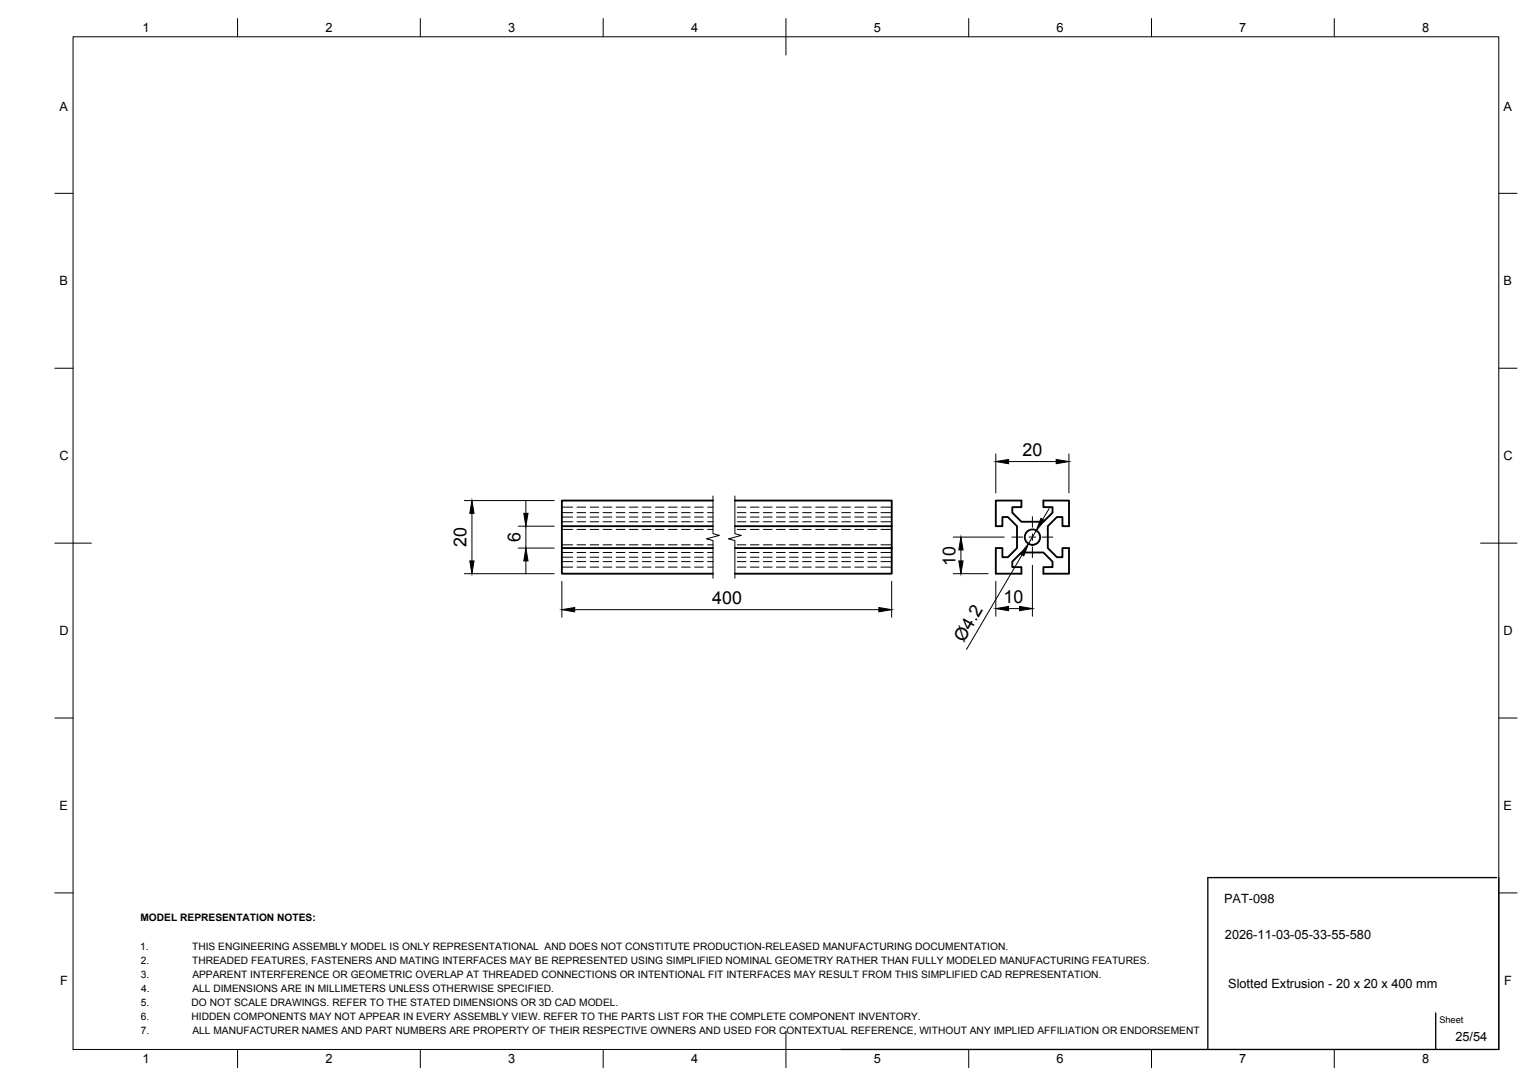
ISO-10303-21;
HEADER;
/* Generated by software containing ST-Developer
 * from STEP Tools, Inc. (www.steptools.com) 
 */

FILE_DESCRIPTION(
/* description */ ('Spring compression tester'),
/* implementation_level */ '2;1');

FILE_NAME(
/* name */ 'Slotted Extrusion - 20 x 20 x 400 mm.step',
/* time_stamp */ '2026-10-28T03:24:11-07:00',
/* author */ (''),
/* organization */ (''),
/* preprocessor_version */ 'ST-DEVELOPER v20.2',
/* originating_system */ 'Autodesk Translation Framework v15.17.0.0',
/* authorisation */ '');

FILE_SCHEMA (('AUTOMOTIVE_DESIGN { 1 0 10303 214 3 1 1 }'));
ENDSEC;

DATA;
#10=MECHANICAL_DESIGN_GEOMETRIC_PRESENTATION_REPRESENTATION('',(#1154),#43521);
#1019=SHAPE_REPRESENTATION_RELATIONSHIP('SRR','None',#43833,#1079);
#1079=ADVANCED_BREP_SHAPE_REPRESENTATION('',(#1226),#43493);
#1154=STYLED_ITEM('',(#44188),#1226);
#1226=MANIFOLD_SOLID_BREP('Body1',#18594);
#1471=FACE_BOUND('',#4046,.T.);
#1472=FACE_BOUND('',#4048,.T.);
#1944=PLANE('',#20307);
#1945=PLANE('',#20308);
#1946=PLANE('',#20309);
#1947=PLANE('',#20310);
#1948=PLANE('',#20311);
#1949=PLANE('',#20312);
#1950=PLANE('',#20313);
#1951=PLANE('',#20314);
#1952=PLANE('',#20315);
#1953=PLANE('',#20316);
#1954=PLANE('',#20317);
#1955=PLANE('',#20318);
#1956=PLANE('',#20319);
#1957=PLANE('',#20320);
#1958=PLANE('',#20321);
#1959=PLANE('',#20322);
#1960=PLANE('',#20323);
#1961=PLANE('',#20324);
#1962=PLANE('',#20325);
#1963=PLANE('',#20326);
#1964=PLANE('',#20327);
#1965=PLANE('',#20328);
#1966=PLANE('',#20329);
#1967=PLANE('',#20330);
#1968=PLANE('',#20331);
#1969=PLANE('',#20332);
#1970=PLANE('',#20333);
#1971=PLANE('',#20334);
#1972=PLANE('',#20335);
#1973=PLANE('',#20336);
#1974=PLANE('',#20337);
#1975=PLANE('',#20338);
#1976=PLANE('',#20339);
#1977=PLANE('',#20340);
#1978=PLANE('',#20341);
#1979=PLANE('',#20342);
#1980=PLANE('',#20346);
#1981=PLANE('',#20347);
#1982=PLANE('',#20348);
#1983=PLANE('',#20349);
#1984=PLANE('',#20350);
#1985=PLANE('',#20351);
#1986=PLANE('',#20352);
#1987=PLANE('',#20353);
#1988=PLANE('',#20354);
#1989=PLANE('',#20355);
#2729=FACE_OUTER_BOUND('',#4000,.T.);
#2730=FACE_OUTER_BOUND('',#4001,.T.);
#2731=FACE_OUTER_BOUND('',#4002,.T.);
#2732=FACE_OUTER_BOUND('',#4003,.T.);
#2733=FACE_OUTER_BOUND('',#4004,.T.);
#2734=FACE_OUTER_BOUND('',#4005,.T.);
#2735=FACE_OUTER_BOUND('',#4006,.T.);
#2736=FACE_OUTER_BOUND('',#4007,.T.);
#2737=FACE_OUTER_BOUND('',#4008,.T.);
#2738=FACE_OUTER_BOUND('',#4009,.T.);
#2739=FACE_OUTER_BOUND('',#4010,.T.);
#2740=FACE_OUTER_BOUND('',#4011,.T.);
#2741=FACE_OUTER_BOUND('',#4012,.T.);
#2742=FACE_OUTER_BOUND('',#4013,.T.);
#2743=FACE_OUTER_BOUND('',#4014,.T.);
#2744=FACE_OUTER_BOUND('',#4015,.T.);
#2745=FACE_OUTER_BOUND('',#4016,.T.);
#2746=FACE_OUTER_BOUND('',#4017,.T.);
#2747=FACE_OUTER_BOUND('',#4018,.T.);
#2748=FACE_OUTER_BOUND('',#4019,.T.);
#2749=FACE_OUTER_BOUND('',#4020,.T.);
#2750=FACE_OUTER_BOUND('',#4021,.T.);
#2751=FACE_OUTER_BOUND('',#4022,.T.);
#2752=FACE_OUTER_BOUND('',#4023,.T.);
#2753=FACE_OUTER_BOUND('',#4024,.T.);
#2754=FACE_OUTER_BOUND('',#4025,.T.);
#2755=FACE_OUTER_BOUND('',#4026,.T.);
#2756=FACE_OUTER_BOUND('',#4027,.T.);
#2757=FACE_OUTER_BOUND('',#4028,.T.);
#2758=FACE_OUTER_BOUND('',#4029,.T.);
#2759=FACE_OUTER_BOUND('',#4030,.T.);
#2760=FACE_OUTER_BOUND('',#4031,.T.);
#2761=FACE_OUTER_BOUND('',#4032,.T.);
#2762=FACE_OUTER_BOUND('',#4033,.T.);
#2763=FACE_OUTER_BOUND('',#4034,.T.);
#2764=FACE_OUTER_BOUND('',#4035,.T.);
#2765=FACE_OUTER_BOUND('',#4036,.T.);
#2766=FACE_OUTER_BOUND('',#4037,.T.);
#2767=FACE_OUTER_BOUND('',#4038,.T.);
#2768=FACE_OUTER_BOUND('',#4039,.T.);
#2769=FACE_OUTER_BOUND('',#4040,.T.);
#2770=FACE_OUTER_BOUND('',#4041,.T.);
#2771=FACE_OUTER_BOUND('',#4042,.T.);
#2772=FACE_OUTER_BOUND('',#4043,.T.);
#2773=FACE_OUTER_BOUND('',#4044,.T.);
#2774=FACE_OUTER_BOUND('',#4045,.T.);
#2775=FACE_OUTER_BOUND('',#4047,.T.);
#4000=EDGE_LOOP('',(#14657,#14658,#14659,#14660));
#4001=EDGE_LOOP('',(#14661,#14662,#14663,#14664));
#4002=EDGE_LOOP('',(#14665,#14666,#14667,#14668));
#4003=EDGE_LOOP('',(#14669,#14670,#14671,#14672));
#4004=EDGE_LOOP('',(#14673,#14674,#14675,#14676));
#4005=EDGE_LOOP('',(#14677,#14678,#14679,#14680));
#4006=EDGE_LOOP('',(#14681,#14682,#14683,#14684));
#4007=EDGE_LOOP('',(#14685,#14686,#14687,#14688));
#4008=EDGE_LOOP('',(#14689,#14690,#14691,#14692));
#4009=EDGE_LOOP('',(#14693,#14694,#14695,#14696));
#4010=EDGE_LOOP('',(#14697,#14698,#14699,#14700));
#4011=EDGE_LOOP('',(#14701,#14702,#14703,#14704));
#4012=EDGE_LOOP('',(#14705,#14706,#14707,#14708));
#4013=EDGE_LOOP('',(#14709,#14710,#14711,#14712));
#4014=EDGE_LOOP('',(#14713,#14714,#14715,#14716));
#4015=EDGE_LOOP('',(#14717,#14718,#14719,#14720));
#4016=EDGE_LOOP('',(#14721,#14722,#14723,#14724));
#4017=EDGE_LOOP('',(#14725,#14726,#14727,#14728));
#4018=EDGE_LOOP('',(#14729,#14730,#14731,#14732));
#4019=EDGE_LOOP('',(#14733,#14734,#14735,#14736));
#4020=EDGE_LOOP('',(#14737,#14738,#14739,#14740));
#4021=EDGE_LOOP('',(#14741,#14742,#14743,#14744));
#4022=EDGE_LOOP('',(#14745,#14746,#14747,#14748));
#4023=EDGE_LOOP('',(#14749,#14750,#14751,#14752));
#4024=EDGE_LOOP('',(#14753,#14754,#14755,#14756));
#4025=EDGE_LOOP('',(#14757,#14758,#14759,#14760));
#4026=EDGE_LOOP('',(#14761,#14762,#14763,#14764));
#4027=EDGE_LOOP('',(#14765,#14766,#14767,#14768));
#4028=EDGE_LOOP('',(#14769,#14770,#14771,#14772));
#4029=EDGE_LOOP('',(#14773,#14774,#14775,#14776));
#4030=EDGE_LOOP('',(#14777,#14778,#14779,#14780));
#4031=EDGE_LOOP('',(#14781,#14782,#14783,#14784));
#4032=EDGE_LOOP('',(#14785,#14786,#14787,#14788));
#4033=EDGE_LOOP('',(#14789,#14790,#14791,#14792));
#4034=EDGE_LOOP('',(#14793,#14794,#14795,#14796));
#4035=EDGE_LOOP('',(#14797,#14798,#14799,#14800));
#4036=EDGE_LOOP('',(#14801,#14802,#14803,#14804));
#4037=EDGE_LOOP('',(#14805,#14806,#14807,#14808));
#4038=EDGE_LOOP('',(#14809,#14810,#14811,#14812));
#4039=EDGE_LOOP('',(#14813,#14814,#14815,#14816));
#4040=EDGE_LOOP('',(#14817,#14818,#14819,#14820));
#4041=EDGE_LOOP('',(#14821,#14822,#14823,#14824));
#4042=EDGE_LOOP('',(#14825,#14826,#14827,#14828));
#4043=EDGE_LOOP('',(#14829,#14830,#14831,#14832));
#4044=EDGE_LOOP('',(#14833,#14834,#14835,#14836));
#4045=EDGE_LOOP('',(#14837,#14838,#14839,#14840,#14841,#14842,#14843,#14844,
#14845,#14846,#14847,#14848,#14849,#14850,#14851,#14852,#14853,#14854,#14855,
#14856,#14857,#14858,#14859,#14860,#14861,#14862,#14863,#14864,#14865,#14866,
#14867,#14868,#14869,#14870,#14871,#14872,#14873,#14874,#14875,#14876,#14877,
#14878,#14879,#14880));
#4046=EDGE_LOOP('',(#14881));
#4047=EDGE_LOOP('',(#14882,#14883,#14884,#14885,#14886,#14887,#14888,#14889,
#14890,#14891,#14892,#14893,#14894,#14895,#14896,#14897,#14898,#14899,#14900,
#14901,#14902,#14903,#14904,#14905,#14906,#14907,#14908,#14909,#14910,#14911,
#14912,#14913,#14914,#14915,#14916,#14917,#14918,#14919,#14920,#14921,#14922,
#14923,#14924,#14925));
#4048=EDGE_LOOP('',(#14926));
#5380=LINE('',#29743,#6812);
#5381=LINE('',#29745,#6813);
#5382=LINE('',#29747,#6814);
#5383=LINE('',#29748,#6815);
#5384=LINE('',#29751,#6816);
#5385=LINE('',#29753,#6817);
#5386=LINE('',#29754,#6818);
#5387=LINE('',#29757,#6819);
#5388=LINE('',#29759,#6820);
#5389=LINE('',#29760,#6821);
#5390=LINE('',#29763,#6822);
#5391=LINE('',#29765,#6823);
#5392=LINE('',#29766,#6824);
#5393=LINE('',#29769,#6825);
#5394=LINE('',#29771,#6826);
#5395=LINE('',#29772,#6827);
#5396=LINE('',#29775,#6828);
#5397=LINE('',#29777,#6829);
#5398=LINE('',#29778,#6830);
#5399=LINE('',#29781,#6831);
#5400=LINE('',#29783,#6832);
#5401=LINE('',#29784,#6833);
#5402=LINE('',#29787,#6834);
#5403=LINE('',#29789,#6835);
#5404=LINE('',#29790,#6836);
#5405=LINE('',#29793,#6837);
#5406=LINE('',#29795,#6838);
#5407=LINE('',#29796,#6839);
#5408=LINE('',#29800,#6840);
#5409=LINE('',#29802,#6841);
#5410=LINE('',#29804,#6842);
#5411=LINE('',#29805,#6843);
#5412=LINE('',#29808,#6844);
#5413=LINE('',#29810,#6845);
#5414=LINE('',#29811,#6846);
#5415=LINE('',#29814,#6847);
#5416=LINE('',#29816,#6848);
#5417=LINE('',#29817,#6849);
#5418=LINE('',#29820,#6850);
#5419=LINE('',#29822,#6851);
#5420=LINE('',#29823,#6852);
#5421=LINE('',#29826,#6853);
#5422=LINE('',#29828,#6854);
#5423=LINE('',#29829,#6855);
#5424=LINE('',#29832,#6856);
#5425=LINE('',#29834,#6857);
#5426=LINE('',#29835,#6858);
#5427=LINE('',#29838,#6859);
#5428=LINE('',#29840,#6860);
#5429=LINE('',#29841,#6861);
#5430=LINE('',#29844,#6862);
#5431=LINE('',#29846,#6863);
#5432=LINE('',#29847,#6864);
#5433=LINE('',#29850,#6865);
#5434=LINE('',#29852,#6866);
#5435=LINE('',#29853,#6867);
#5436=LINE('',#29857,#6868);
#5437=LINE('',#29859,#6869);
#5438=LINE('',#29861,#6870);
#5439=LINE('',#29862,#6871);
#5440=LINE('',#29865,#6872);
#5441=LINE('',#29867,#6873);
#5442=LINE('',#29868,#6874);
#5443=LINE('',#29871,#6875);
#5444=LINE('',#29873,#6876);
#5445=LINE('',#29874,#6877);
#5446=LINE('',#29877,#6878);
#5447=LINE('',#29879,#6879);
#5448=LINE('',#29880,#6880);
#5449=LINE('',#29883,#6881);
#5450=LINE('',#29885,#6882);
#5451=LINE('',#29886,#6883);
#5452=LINE('',#29889,#6884);
#5453=LINE('',#29891,#6885);
#5454=LINE('',#29892,#6886);
#5455=LINE('',#29895,#6887);
#5456=LINE('',#29897,#6888);
#5457=LINE('',#29898,#6889);
#5458=LINE('',#29901,#6890);
#5459=LINE('',#29903,#6891);
#5460=LINE('',#29904,#6892);
#5461=LINE('',#29907,#6893);
#5462=LINE('',#29909,#6894);
#5463=LINE('',#29910,#6895);
#5464=LINE('',#29914,#6896);
#5465=LINE('',#29916,#6897);
#5466=LINE('',#29918,#6898);
#5467=LINE('',#29919,#6899);
#5468=LINE('',#29922,#6900);
#5469=LINE('',#29924,#6901);
#5470=LINE('',#29925,#6902);
#5471=LINE('',#29928,#6903);
#5472=LINE('',#29930,#6904);
#5473=LINE('',#29931,#6905);
#5474=LINE('',#29934,#6906);
#5475=LINE('',#29936,#6907);
#5476=LINE('',#29937,#6908);
#5477=LINE('',#29940,#6909);
#5478=LINE('',#29942,#6910);
#5479=LINE('',#29943,#6911);
#5480=LINE('',#29946,#6912);
#5481=LINE('',#29948,#6913);
#5482=LINE('',#29949,#6914);
#5483=LINE('',#29952,#6915);
#5484=LINE('',#29954,#6916);
#5485=LINE('',#29955,#6917);
#5486=LINE('',#29958,#6918);
#5487=LINE('',#29960,#6919);
#5488=LINE('',#29961,#6920);
#5489=LINE('',#29964,#6921);
#5490=LINE('',#29966,#6922);
#5491=LINE('',#29967,#6923);
#5492=LINE('',#29972,#6924);
#5493=LINE('',#29976,#6925);
#5494=LINE('',#29978,#6926);
#5495=LINE('',#29979,#6927);
#5496=LINE('',#29982,#6928);
#5497=LINE('',#29984,#6929);
#5498=LINE('',#29985,#6930);
#5499=LINE('',#29987,#6931);
#5500=LINE('',#29988,#6932);
#5501=LINE('',#29991,#6933);
#5502=LINE('',#29993,#6934);
#5503=LINE('',#29994,#6935);
#5504=LINE('',#29996,#6936);
#5505=LINE('',#29997,#6937);
#5506=LINE('',#30000,#6938);
#5507=LINE('',#30002,#6939);
#5508=LINE('',#30003,#6940);
#5509=LINE('',#30005,#6941);
#5510=LINE('',#30006,#6942);
#5511=LINE('',#30008,#6943);
#5512=LINE('',#30009,#6944);
#6812=VECTOR('',#24018,1.);
#6813=VECTOR('',#24019,1.);
#6814=VECTOR('',#24020,1.);
#6815=VECTOR('',#24021,1.);
#6816=VECTOR('',#24024,1.);
#6817=VECTOR('',#24025,1.);
#6818=VECTOR('',#24026,1.);
#6819=VECTOR('',#24029,1.);
#6820=VECTOR('',#24030,1.);
#6821=VECTOR('',#24031,1.);
#6822=VECTOR('',#24034,1.);
#6823=VECTOR('',#24035,1.);
#6824=VECTOR('',#24036,1.);
#6825=VECTOR('',#24039,1.);
#6826=VECTOR('',#24040,1.);
#6827=VECTOR('',#24041,1.);
#6828=VECTOR('',#24044,1.);
#6829=VECTOR('',#24045,1.);
#6830=VECTOR('',#24046,1.);
#6831=VECTOR('',#24049,1.);
#6832=VECTOR('',#24050,1.);
#6833=VECTOR('',#24051,1.);
#6834=VECTOR('',#24054,1.);
#6835=VECTOR('',#24055,1.);
#6836=VECTOR('',#24056,1.);
#6837=VECTOR('',#24059,1.);
#6838=VECTOR('',#24060,1.);
#6839=VECTOR('',#24061,1.);
#6840=VECTOR('',#24064,1.);
#6841=VECTOR('',#24065,1.);
#6842=VECTOR('',#24066,1.);
#6843=VECTOR('',#24067,1.);
#6844=VECTOR('',#24070,1.);
#6845=VECTOR('',#24071,1.);
#6846=VECTOR('',#24072,1.);
#6847=VECTOR('',#24075,1.);
#6848=VECTOR('',#24076,1.);
#6849=VECTOR('',#24077,1.);
#6850=VECTOR('',#24080,1.);
#6851=VECTOR('',#24081,1.);
#6852=VECTOR('',#24082,1.);
#6853=VECTOR('',#24085,1.);
#6854=VECTOR('',#24086,1.);
#6855=VECTOR('',#24087,1.);
#6856=VECTOR('',#24090,1.);
#6857=VECTOR('',#24091,1.);
#6858=VECTOR('',#24092,1.);
#6859=VECTOR('',#24095,1.);
#6860=VECTOR('',#24096,1.);
#6861=VECTOR('',#24097,1.);
#6862=VECTOR('',#24100,1.);
#6863=VECTOR('',#24101,1.);
#6864=VECTOR('',#24102,1.);
#6865=VECTOR('',#24105,1.);
#6866=VECTOR('',#24106,1.);
#6867=VECTOR('',#24107,1.);
#6868=VECTOR('',#24110,1.);
#6869=VECTOR('',#24111,1.);
#6870=VECTOR('',#24112,1.);
#6871=VECTOR('',#24113,1.);
#6872=VECTOR('',#24116,1.);
#6873=VECTOR('',#24117,1.);
#6874=VECTOR('',#24118,1.);
#6875=VECTOR('',#24121,1.);
#6876=VECTOR('',#24122,1.);
#6877=VECTOR('',#24123,1.);
#6878=VECTOR('',#24126,1.);
#6879=VECTOR('',#24127,1.);
#6880=VECTOR('',#24128,1.);
#6881=VECTOR('',#24131,1.);
#6882=VECTOR('',#24132,1.);
#6883=VECTOR('',#24133,1.);
#6884=VECTOR('',#24136,1.);
#6885=VECTOR('',#24137,1.);
#6886=VECTOR('',#24138,1.);
#6887=VECTOR('',#24141,1.);
#6888=VECTOR('',#24142,1.);
#6889=VECTOR('',#24143,1.);
#6890=VECTOR('',#24146,1.);
#6891=VECTOR('',#24147,1.);
#6892=VECTOR('',#24148,1.);
#6893=VECTOR('',#24151,1.);
#6894=VECTOR('',#24152,1.);
#6895=VECTOR('',#24153,1.);
#6896=VECTOR('',#24156,1.);
#6897=VECTOR('',#24157,1.);
#6898=VECTOR('',#24158,1.);
#6899=VECTOR('',#24159,1.);
#6900=VECTOR('',#24162,1.);
#6901=VECTOR('',#24163,1.);
#6902=VECTOR('',#24164,1.);
#6903=VECTOR('',#24167,1.);
#6904=VECTOR('',#24168,1.);
#6905=VECTOR('',#24169,1.);
#6906=VECTOR('',#24172,1.);
#6907=VECTOR('',#24173,1.);
#6908=VECTOR('',#24174,1.);
#6909=VECTOR('',#24177,1.);
#6910=VECTOR('',#24178,1.);
#6911=VECTOR('',#24179,1.);
#6912=VECTOR('',#24182,1.);
#6913=VECTOR('',#24183,1.);
#6914=VECTOR('',#24184,1.);
#6915=VECTOR('',#24187,1.);
#6916=VECTOR('',#24188,1.);
#6917=VECTOR('',#24189,1.);
#6918=VECTOR('',#24192,1.);
#6919=VECTOR('',#24193,1.);
#6920=VECTOR('',#24194,1.);
#6921=VECTOR('',#24197,1.);
#6922=VECTOR('',#24198,1.);
#6923=VECTOR('',#24199,1.);
#6924=VECTOR('',#24204,0.21);
#6925=VECTOR('',#24209,1.);
#6926=VECTOR('',#24210,1.);
#6927=VECTOR('',#24211,1.);
#6928=VECTOR('',#24214,1.);
#6929=VECTOR('',#24215,1.);
#6930=VECTOR('',#24216,1.);
#6931=VECTOR('',#24219,1.);
#6932=VECTOR('',#24220,1.);
#6933=VECTOR('',#24223,1.);
#6934=VECTOR('',#24224,1.);
#6935=VECTOR('',#24225,1.);
#6936=VECTOR('',#24228,1.);
#6937=VECTOR('',#24229,1.);
#6938=VECTOR('',#24232,1.);
#6939=VECTOR('',#24233,1.);
#6940=VECTOR('',#24234,1.);
#6941=VECTOR('',#24237,1.);
#6942=VECTOR('',#24238,1.);
#6943=VECTOR('',#24241,1.);
#6944=VECTOR('',#24242,1.);
#7884=CIRCLE('',#20344,0.21);
#7885=CIRCLE('',#20345,0.21);
#8963=VERTEX_POINT('',#29741);
#8964=VERTEX_POINT('',#29742);
#8965=VERTEX_POINT('',#29744);
#8966=VERTEX_POINT('',#29746);
#8967=VERTEX_POINT('',#29750);
#8968=VERTEX_POINT('',#29752);
#8969=VERTEX_POINT('',#29756);
#8970=VERTEX_POINT('',#29758);
#8971=VERTEX_POINT('',#29762);
#8972=VERTEX_POINT('',#29764);
#8973=VERTEX_POINT('',#29768);
#8974=VERTEX_POINT('',#29770);
#8975=VERTEX_POINT('',#29774);
#8976=VERTEX_POINT('',#29776);
#8977=VERTEX_POINT('',#29780);
#8978=VERTEX_POINT('',#29782);
#8979=VERTEX_POINT('',#29786);
#8980=VERTEX_POINT('',#29788);
#8981=VERTEX_POINT('',#29792);
#8982=VERTEX_POINT('',#29794);
#8983=VERTEX_POINT('',#29798);
#8984=VERTEX_POINT('',#29799);
#8985=VERTEX_POINT('',#29801);
#8986=VERTEX_POINT('',#29803);
#8987=VERTEX_POINT('',#29807);
#8988=VERTEX_POINT('',#29809);
#8989=VERTEX_POINT('',#29813);
#8990=VERTEX_POINT('',#29815);
#8991=VERTEX_POINT('',#29819);
#8992=VERTEX_POINT('',#29821);
#8993=VERTEX_POINT('',#29825);
#8994=VERTEX_POINT('',#29827);
#8995=VERTEX_POINT('',#29831);
#8996=VERTEX_POINT('',#29833);
#8997=VERTEX_POINT('',#29837);
#8998=VERTEX_POINT('',#29839);
#8999=VERTEX_POINT('',#29843);
#9000=VERTEX_POINT('',#29845);
#9001=VERTEX_POINT('',#29849);
#9002=VERTEX_POINT('',#29851);
#9003=VERTEX_POINT('',#29855);
#9004=VERTEX_POINT('',#29856);
#9005=VERTEX_POINT('',#29858);
#9006=VERTEX_POINT('',#29860);
#9007=VERTEX_POINT('',#29864);
#9008=VERTEX_POINT('',#29866);
#9009=VERTEX_POINT('',#29870);
#9010=VERTEX_POINT('',#29872);
#9011=VERTEX_POINT('',#29876);
#9012=VERTEX_POINT('',#29878);
#9013=VERTEX_POINT('',#29882);
#9014=VERTEX_POINT('',#29884);
#9015=VERTEX_POINT('',#29888);
#9016=VERTEX_POINT('',#29890);
#9017=VERTEX_POINT('',#29894);
#9018=VERTEX_POINT('',#29896);
#9019=VERTEX_POINT('',#29900);
#9020=VERTEX_POINT('',#29902);
#9021=VERTEX_POINT('',#29906);
#9022=VERTEX_POINT('',#29908);
#9023=VERTEX_POINT('',#29912);
#9024=VERTEX_POINT('',#29913);
#9025=VERTEX_POINT('',#29915);
#9026=VERTEX_POINT('',#29917);
#9027=VERTEX_POINT('',#29921);
#9028=VERTEX_POINT('',#29923);
#9029=VERTEX_POINT('',#29927);
#9030=VERTEX_POINT('',#29929);
#9031=VERTEX_POINT('',#29933);
#9032=VERTEX_POINT('',#29935);
#9033=VERTEX_POINT('',#29939);
#9034=VERTEX_POINT('',#29941);
#9035=VERTEX_POINT('',#29945);
#9036=VERTEX_POINT('',#29947);
#9037=VERTEX_POINT('',#29951);
#9038=VERTEX_POINT('',#29953);
#9039=VERTEX_POINT('',#29957);
#9040=VERTEX_POINT('',#29959);
#9041=VERTEX_POINT('',#29963);
#9042=VERTEX_POINT('',#29965);
#9043=VERTEX_POINT('',#29969);
#9044=VERTEX_POINT('',#29971);
#9045=VERTEX_POINT('',#29975);
#9046=VERTEX_POINT('',#29977);
#9047=VERTEX_POINT('',#29981);
#9048=VERTEX_POINT('',#29983);
#9049=VERTEX_POINT('',#29990);
#9050=VERTEX_POINT('',#29992);
#9051=VERTEX_POINT('',#29999);
#9052=VERTEX_POINT('',#30001);
#10993=EDGE_CURVE('',#8963,#8964,#5380,.T.);
#10994=EDGE_CURVE('',#8963,#8965,#5381,.T.);
#10995=EDGE_CURVE('',#8966,#8965,#5382,.T.);
#10996=EDGE_CURVE('',#8964,#8966,#5383,.T.);
#10997=EDGE_CURVE('',#8967,#8963,#5384,.T.);
#10998=EDGE_CURVE('',#8967,#8968,#5385,.T.);
#10999=EDGE_CURVE('',#8965,#8968,#5386,.T.);
#11000=EDGE_CURVE('',#8969,#8967,#5387,.T.);
#11001=EDGE_CURVE('',#8969,#8970,#5388,.T.);
#11002=EDGE_CURVE('',#8968,#8970,#5389,.T.);
#11003=EDGE_CURVE('',#8971,#8969,#5390,.T.);
#11004=EDGE_CURVE('',#8971,#8972,#5391,.T.);
#11005=EDGE_CURVE('',#8970,#8972,#5392,.T.);
#11006=EDGE_CURVE('',#8973,#8971,#5393,.T.);
#11007=EDGE_CURVE('',#8973,#8974,#5394,.T.);
#11008=EDGE_CURVE('',#8972,#8974,#5395,.T.);
#11009=EDGE_CURVE('',#8975,#8973,#5396,.T.);
#11010=EDGE_CURVE('',#8975,#8976,#5397,.T.);
#11011=EDGE_CURVE('',#8974,#8976,#5398,.T.);
#11012=EDGE_CURVE('',#8977,#8975,#5399,.T.);
#11013=EDGE_CURVE('',#8977,#8978,#5400,.T.);
#11014=EDGE_CURVE('',#8976,#8978,#5401,.T.);
#11015=EDGE_CURVE('',#8979,#8977,#5402,.T.);
#11016=EDGE_CURVE('',#8979,#8980,#5403,.T.);
#11017=EDGE_CURVE('',#8978,#8980,#5404,.T.);
#11018=EDGE_CURVE('',#8981,#8979,#5405,.T.);
#11019=EDGE_CURVE('',#8982,#8981,#5406,.T.);
#11020=EDGE_CURVE('',#8980,#8982,#5407,.T.);
#11021=EDGE_CURVE('',#8983,#8984,#5408,.T.);
#11022=EDGE_CURVE('',#8983,#8985,#5409,.T.);
#11023=EDGE_CURVE('',#8986,#8985,#5410,.T.);
#11024=EDGE_CURVE('',#8984,#8986,#5411,.T.);
#11025=EDGE_CURVE('',#8987,#8983,#5412,.T.);
#11026=EDGE_CURVE('',#8987,#8988,#5413,.T.);
#11027=EDGE_CURVE('',#8985,#8988,#5414,.T.);
#11028=EDGE_CURVE('',#8989,#8987,#5415,.T.);
#11029=EDGE_CURVE('',#8989,#8990,#5416,.T.);
#11030=EDGE_CURVE('',#8988,#8990,#5417,.T.);
#11031=EDGE_CURVE('',#8991,#8989,#5418,.T.);
#11032=EDGE_CURVE('',#8991,#8992,#5419,.T.);
#11033=EDGE_CURVE('',#8990,#8992,#5420,.T.);
#11034=EDGE_CURVE('',#8993,#8991,#5421,.T.);
#11035=EDGE_CURVE('',#8993,#8994,#5422,.T.);
#11036=EDGE_CURVE('',#8992,#8994,#5423,.T.);
#11037=EDGE_CURVE('',#8995,#8993,#5424,.T.);
#11038=EDGE_CURVE('',#8995,#8996,#5425,.T.);
#11039=EDGE_CURVE('',#8994,#8996,#5426,.T.);
#11040=EDGE_CURVE('',#8997,#8995,#5427,.T.);
#11041=EDGE_CURVE('',#8997,#8998,#5428,.T.);
#11042=EDGE_CURVE('',#8996,#8998,#5429,.T.);
#11043=EDGE_CURVE('',#8999,#8997,#5430,.T.);
#11044=EDGE_CURVE('',#8999,#9000,#5431,.T.);
#11045=EDGE_CURVE('',#8998,#9000,#5432,.T.);
#11046=EDGE_CURVE('',#9001,#8999,#5433,.T.);
#11047=EDGE_CURVE('',#9002,#9001,#5434,.T.);
#11048=EDGE_CURVE('',#9000,#9002,#5435,.T.);
#11049=EDGE_CURVE('',#9003,#9004,#5436,.T.);
#11050=EDGE_CURVE('',#9003,#9005,#5437,.T.);
#11051=EDGE_CURVE('',#9006,#9005,#5438,.T.);
#11052=EDGE_CURVE('',#9004,#9006,#5439,.T.);
#11053=EDGE_CURVE('',#9007,#9003,#5440,.T.);
#11054=EDGE_CURVE('',#9007,#9008,#5441,.T.);
#11055=EDGE_CURVE('',#9005,#9008,#5442,.T.);
#11056=EDGE_CURVE('',#9009,#9007,#5443,.T.);
#11057=EDGE_CURVE('',#9009,#9010,#5444,.T.);
#11058=EDGE_CURVE('',#9008,#9010,#5445,.T.);
#11059=EDGE_CURVE('',#9011,#9009,#5446,.T.);
#11060=EDGE_CURVE('',#9011,#9012,#5447,.T.);
#11061=EDGE_CURVE('',#9010,#9012,#5448,.T.);
#11062=EDGE_CURVE('',#9013,#9011,#5449,.T.);
#11063=EDGE_CURVE('',#9013,#9014,#5450,.T.);
#11064=EDGE_CURVE('',#9012,#9014,#5451,.T.);
#11065=EDGE_CURVE('',#9015,#9013,#5452,.T.);
#11066=EDGE_CURVE('',#9015,#9016,#5453,.T.);
#11067=EDGE_CURVE('',#9014,#9016,#5454,.T.);
#11068=EDGE_CURVE('',#9017,#9015,#5455,.T.);
#11069=EDGE_CURVE('',#9017,#9018,#5456,.T.);
#11070=EDGE_CURVE('',#9016,#9018,#5457,.T.);
#11071=EDGE_CURVE('',#9019,#9017,#5458,.T.);
#11072=EDGE_CURVE('',#9019,#9020,#5459,.T.);
#11073=EDGE_CURVE('',#9018,#9020,#5460,.T.);
#11074=EDGE_CURVE('',#9021,#9019,#5461,.T.);
#11075=EDGE_CURVE('',#9022,#9021,#5462,.T.);
#11076=EDGE_CURVE('',#9020,#9022,#5463,.T.);
#11077=EDGE_CURVE('',#9023,#9024,#5464,.T.);
#11078=EDGE_CURVE('',#9023,#9025,#5465,.T.);
#11079=EDGE_CURVE('',#9026,#9025,#5466,.T.);
#11080=EDGE_CURVE('',#9024,#9026,#5467,.T.);
#11081=EDGE_CURVE('',#9027,#9023,#5468,.T.);
#11082=EDGE_CURVE('',#9027,#9028,#5469,.T.);
#11083=EDGE_CURVE('',#9025,#9028,#5470,.T.);
#11084=EDGE_CURVE('',#9029,#9027,#5471,.T.);
#11085=EDGE_CURVE('',#9029,#9030,#5472,.T.);
#11086=EDGE_CURVE('',#9028,#9030,#5473,.T.);
#11087=EDGE_CURVE('',#9031,#9029,#5474,.T.);
#11088=EDGE_CURVE('',#9031,#9032,#5475,.T.);
#11089=EDGE_CURVE('',#9030,#9032,#5476,.T.);
#11090=EDGE_CURVE('',#9033,#9031,#5477,.T.);
#11091=EDGE_CURVE('',#9033,#9034,#5478,.T.);
#11092=EDGE_CURVE('',#9032,#9034,#5479,.T.);
#11093=EDGE_CURVE('',#9035,#9033,#5480,.T.);
#11094=EDGE_CURVE('',#9035,#9036,#5481,.T.);
#11095=EDGE_CURVE('',#9034,#9036,#5482,.T.);
#11096=EDGE_CURVE('',#9037,#9035,#5483,.T.);
#11097=EDGE_CURVE('',#9037,#9038,#5484,.T.);
#11098=EDGE_CURVE('',#9036,#9038,#5485,.T.);
#11099=EDGE_CURVE('',#9039,#9037,#5486,.T.);
#11100=EDGE_CURVE('',#9039,#9040,#5487,.T.);
#11101=EDGE_CURVE('',#9038,#9040,#5488,.T.);
#11102=EDGE_CURVE('',#9041,#9039,#5489,.T.);
#11103=EDGE_CURVE('',#9042,#9041,#5490,.T.);
#11104=EDGE_CURVE('',#9040,#9042,#5491,.T.);
#11105=EDGE_CURVE('',#9043,#9043,#7884,.T.);
#11106=EDGE_CURVE('',#9043,#9044,#5492,.T.);
#11107=EDGE_CURVE('',#9044,#9044,#7885,.T.);
#11108=EDGE_CURVE('',#8981,#9045,#5493,.T.);
#11109=EDGE_CURVE('',#9045,#9046,#5494,.T.);
#11110=EDGE_CURVE('',#8982,#9046,#5495,.T.);
#11111=EDGE_CURVE('',#9047,#8966,#5496,.T.);
#11112=EDGE_CURVE('',#9048,#9047,#5497,.T.);
#11113=EDGE_CURVE('',#9048,#8964,#5498,.T.);
#11114=EDGE_CURVE('',#9001,#9048,#5499,.T.);
#11115=EDGE_CURVE('',#9002,#9047,#5500,.T.);
#11116=EDGE_CURVE('',#9049,#8986,#5501,.T.);
#11117=EDGE_CURVE('',#9050,#9049,#5502,.T.);
#11118=EDGE_CURVE('',#9050,#8984,#5503,.T.);
#11119=EDGE_CURVE('',#9021,#9050,#5504,.T.);
#11120=EDGE_CURVE('',#9022,#9049,#5505,.T.);
#11121=EDGE_CURVE('',#9051,#9006,#5506,.T.);
#11122=EDGE_CURVE('',#9052,#9051,#5507,.T.);
#11123=EDGE_CURVE('',#9052,#9004,#5508,.T.);
#11124=EDGE_CURVE('',#9041,#9052,#5509,.T.);
#11125=EDGE_CURVE('',#9042,#9051,#5510,.T.);
#11126=EDGE_CURVE('',#9046,#9026,#5511,.T.);
#11127=EDGE_CURVE('',#9045,#9024,#5512,.T.);
#14657=ORIENTED_EDGE('',*,*,#10993,.F.);
#14658=ORIENTED_EDGE('',*,*,#10994,.T.);
#14659=ORIENTED_EDGE('',*,*,#10995,.F.);
#14660=ORIENTED_EDGE('',*,*,#10996,.F.);
#14661=ORIENTED_EDGE('',*,*,#10997,.F.);
#14662=ORIENTED_EDGE('',*,*,#10998,.T.);
#14663=ORIENTED_EDGE('',*,*,#10999,.F.);
#14664=ORIENTED_EDGE('',*,*,#10994,.F.);
#14665=ORIENTED_EDGE('',*,*,#11000,.F.);
#14666=ORIENTED_EDGE('',*,*,#11001,.T.);
#14667=ORIENTED_EDGE('',*,*,#11002,.F.);
#14668=ORIENTED_EDGE('',*,*,#10998,.F.);
#14669=ORIENTED_EDGE('',*,*,#11003,.F.);
#14670=ORIENTED_EDGE('',*,*,#11004,.T.);
#14671=ORIENTED_EDGE('',*,*,#11005,.F.);
#14672=ORIENTED_EDGE('',*,*,#11001,.F.);
#14673=ORIENTED_EDGE('',*,*,#11006,.F.);
#14674=ORIENTED_EDGE('',*,*,#11007,.T.);
#14675=ORIENTED_EDGE('',*,*,#11008,.F.);
#14676=ORIENTED_EDGE('',*,*,#11004,.F.);
#14677=ORIENTED_EDGE('',*,*,#11009,.F.);
#14678=ORIENTED_EDGE('',*,*,#11010,.T.);
#14679=ORIENTED_EDGE('',*,*,#11011,.F.);
#14680=ORIENTED_EDGE('',*,*,#11007,.F.);
#14681=ORIENTED_EDGE('',*,*,#11012,.F.);
#14682=ORIENTED_EDGE('',*,*,#11013,.T.);
#14683=ORIENTED_EDGE('',*,*,#11014,.F.);
#14684=ORIENTED_EDGE('',*,*,#11010,.F.);
#14685=ORIENTED_EDGE('',*,*,#11015,.F.);
#14686=ORIENTED_EDGE('',*,*,#11016,.T.);
#14687=ORIENTED_EDGE('',*,*,#11017,.F.);
#14688=ORIENTED_EDGE('',*,*,#11013,.F.);
#14689=ORIENTED_EDGE('',*,*,#11018,.F.);
#14690=ORIENTED_EDGE('',*,*,#11019,.F.);
#14691=ORIENTED_EDGE('',*,*,#11020,.F.);
#14692=ORIENTED_EDGE('',*,*,#11016,.F.);
#14693=ORIENTED_EDGE('',*,*,#11021,.F.);
#14694=ORIENTED_EDGE('',*,*,#11022,.T.);
#14695=ORIENTED_EDGE('',*,*,#11023,.F.);
#14696=ORIENTED_EDGE('',*,*,#11024,.F.);
#14697=ORIENTED_EDGE('',*,*,#11025,.F.);
#14698=ORIENTED_EDGE('',*,*,#11026,.T.);
#14699=ORIENTED_EDGE('',*,*,#11027,.F.);
#14700=ORIENTED_EDGE('',*,*,#11022,.F.);
#14701=ORIENTED_EDGE('',*,*,#11028,.F.);
#14702=ORIENTED_EDGE('',*,*,#11029,.T.);
#14703=ORIENTED_EDGE('',*,*,#11030,.F.);
#14704=ORIENTED_EDGE('',*,*,#11026,.F.);
#14705=ORIENTED_EDGE('',*,*,#11031,.F.);
#14706=ORIENTED_EDGE('',*,*,#11032,.T.);
#14707=ORIENTED_EDGE('',*,*,#11033,.F.);
#14708=ORIENTED_EDGE('',*,*,#11029,.F.);
#14709=ORIENTED_EDGE('',*,*,#11034,.F.);
#14710=ORIENTED_EDGE('',*,*,#11035,.T.);
#14711=ORIENTED_EDGE('',*,*,#11036,.F.);
#14712=ORIENTED_EDGE('',*,*,#11032,.F.);
#14713=ORIENTED_EDGE('',*,*,#11037,.F.);
#14714=ORIENTED_EDGE('',*,*,#11038,.T.);
#14715=ORIENTED_EDGE('',*,*,#11039,.F.);
#14716=ORIENTED_EDGE('',*,*,#11035,.F.);
#14717=ORIENTED_EDGE('',*,*,#11040,.F.);
#14718=ORIENTED_EDGE('',*,*,#11041,.T.);
#14719=ORIENTED_EDGE('',*,*,#11042,.F.);
#14720=ORIENTED_EDGE('',*,*,#11038,.F.);
#14721=ORIENTED_EDGE('',*,*,#11043,.F.);
#14722=ORIENTED_EDGE('',*,*,#11044,.T.);
#14723=ORIENTED_EDGE('',*,*,#11045,.F.);
#14724=ORIENTED_EDGE('',*,*,#11041,.F.);
#14725=ORIENTED_EDGE('',*,*,#11046,.F.);
#14726=ORIENTED_EDGE('',*,*,#11047,.F.);
#14727=ORIENTED_EDGE('',*,*,#11048,.F.);
#14728=ORIENTED_EDGE('',*,*,#11044,.F.);
#14729=ORIENTED_EDGE('',*,*,#11049,.F.);
#14730=ORIENTED_EDGE('',*,*,#11050,.T.);
#14731=ORIENTED_EDGE('',*,*,#11051,.F.);
#14732=ORIENTED_EDGE('',*,*,#11052,.F.);
#14733=ORIENTED_EDGE('',*,*,#11053,.F.);
#14734=ORIENTED_EDGE('',*,*,#11054,.T.);
#14735=ORIENTED_EDGE('',*,*,#11055,.F.);
#14736=ORIENTED_EDGE('',*,*,#11050,.F.);
#14737=ORIENTED_EDGE('',*,*,#11056,.F.);
#14738=ORIENTED_EDGE('',*,*,#11057,.T.);
#14739=ORIENTED_EDGE('',*,*,#11058,.F.);
#14740=ORIENTED_EDGE('',*,*,#11054,.F.);
#14741=ORIENTED_EDGE('',*,*,#11059,.F.);
#14742=ORIENTED_EDGE('',*,*,#11060,.T.);
#14743=ORIENTED_EDGE('',*,*,#11061,.F.);
#14744=ORIENTED_EDGE('',*,*,#11057,.F.);
#14745=ORIENTED_EDGE('',*,*,#11062,.F.);
#14746=ORIENTED_EDGE('',*,*,#11063,.T.);
#14747=ORIENTED_EDGE('',*,*,#11064,.F.);
#14748=ORIENTED_EDGE('',*,*,#11060,.F.);
#14749=ORIENTED_EDGE('',*,*,#11065,.F.);
#14750=ORIENTED_EDGE('',*,*,#11066,.T.);
#14751=ORIENTED_EDGE('',*,*,#11067,.F.);
#14752=ORIENTED_EDGE('',*,*,#11063,.F.);
#14753=ORIENTED_EDGE('',*,*,#11068,.F.);
#14754=ORIENTED_EDGE('',*,*,#11069,.T.);
#14755=ORIENTED_EDGE('',*,*,#11070,.F.);
#14756=ORIENTED_EDGE('',*,*,#11066,.F.);
#14757=ORIENTED_EDGE('',*,*,#11071,.F.);
#14758=ORIENTED_EDGE('',*,*,#11072,.T.);
#14759=ORIENTED_EDGE('',*,*,#11073,.F.);
#14760=ORIENTED_EDGE('',*,*,#11069,.F.);
#14761=ORIENTED_EDGE('',*,*,#11074,.F.);
#14762=ORIENTED_EDGE('',*,*,#11075,.F.);
#14763=ORIENTED_EDGE('',*,*,#11076,.F.);
#14764=ORIENTED_EDGE('',*,*,#11072,.F.);
#14765=ORIENTED_EDGE('',*,*,#11077,.F.);
#14766=ORIENTED_EDGE('',*,*,#11078,.T.);
#14767=ORIENTED_EDGE('',*,*,#11079,.F.);
#14768=ORIENTED_EDGE('',*,*,#11080,.F.);
#14769=ORIENTED_EDGE('',*,*,#11081,.F.);
#14770=ORIENTED_EDGE('',*,*,#11082,.T.);
#14771=ORIENTED_EDGE('',*,*,#11083,.F.);
#14772=ORIENTED_EDGE('',*,*,#11078,.F.);
#14773=ORIENTED_EDGE('',*,*,#11084,.F.);
#14774=ORIENTED_EDGE('',*,*,#11085,.T.);
#14775=ORIENTED_EDGE('',*,*,#11086,.F.);
#14776=ORIENTED_EDGE('',*,*,#11082,.F.);
#14777=ORIENTED_EDGE('',*,*,#11087,.F.);
#14778=ORIENTED_EDGE('',*,*,#11088,.T.);
#14779=ORIENTED_EDGE('',*,*,#11089,.F.);
#14780=ORIENTED_EDGE('',*,*,#11085,.F.);
#14781=ORIENTED_EDGE('',*,*,#11090,.F.);
#14782=ORIENTED_EDGE('',*,*,#11091,.T.);
#14783=ORIENTED_EDGE('',*,*,#11092,.F.);
#14784=ORIENTED_EDGE('',*,*,#11088,.F.);
#14785=ORIENTED_EDGE('',*,*,#11093,.F.);
#14786=ORIENTED_EDGE('',*,*,#11094,.T.);
#14787=ORIENTED_EDGE('',*,*,#11095,.F.);
#14788=ORIENTED_EDGE('',*,*,#11091,.F.);
#14789=ORIENTED_EDGE('',*,*,#11096,.F.);
#14790=ORIENTED_EDGE('',*,*,#11097,.T.);
#14791=ORIENTED_EDGE('',*,*,#11098,.F.);
#14792=ORIENTED_EDGE('',*,*,#11094,.F.);
#14793=ORIENTED_EDGE('',*,*,#11099,.F.);
#14794=ORIENTED_EDGE('',*,*,#11100,.T.);
#14795=ORIENTED_EDGE('',*,*,#11101,.F.);
#14796=ORIENTED_EDGE('',*,*,#11097,.F.);
#14797=ORIENTED_EDGE('',*,*,#11102,.F.);
#14798=ORIENTED_EDGE('',*,*,#11103,.F.);
#14799=ORIENTED_EDGE('',*,*,#11104,.F.);
#14800=ORIENTED_EDGE('',*,*,#11100,.F.);
#14801=ORIENTED_EDGE('',*,*,#11105,.F.);
#14802=ORIENTED_EDGE('',*,*,#11106,.T.);
#14803=ORIENTED_EDGE('',*,*,#11107,.F.);
#14804=ORIENTED_EDGE('',*,*,#11106,.F.);
#14805=ORIENTED_EDGE('',*,*,#11019,.T.);
#14806=ORIENTED_EDGE('',*,*,#11108,.T.);
#14807=ORIENTED_EDGE('',*,*,#11109,.T.);
#14808=ORIENTED_EDGE('',*,*,#11110,.F.);
#14809=ORIENTED_EDGE('',*,*,#10996,.T.);
#14810=ORIENTED_EDGE('',*,*,#11111,.F.);
#14811=ORIENTED_EDGE('',*,*,#11112,.F.);
#14812=ORIENTED_EDGE('',*,*,#11113,.T.);
#14813=ORIENTED_EDGE('',*,*,#11047,.T.);
#14814=ORIENTED_EDGE('',*,*,#11114,.T.);
#14815=ORIENTED_EDGE('',*,*,#11112,.T.);
#14816=ORIENTED_EDGE('',*,*,#11115,.F.);
#14817=ORIENTED_EDGE('',*,*,#11024,.T.);
#14818=ORIENTED_EDGE('',*,*,#11116,.F.);
#14819=ORIENTED_EDGE('',*,*,#11117,.F.);
#14820=ORIENTED_EDGE('',*,*,#11118,.T.);
#14821=ORIENTED_EDGE('',*,*,#11075,.T.);
#14822=ORIENTED_EDGE('',*,*,#11119,.T.);
#14823=ORIENTED_EDGE('',*,*,#11117,.T.);
#14824=ORIENTED_EDGE('',*,*,#11120,.F.);
#14825=ORIENTED_EDGE('',*,*,#11052,.T.);
#14826=ORIENTED_EDGE('',*,*,#11121,.F.);
#14827=ORIENTED_EDGE('',*,*,#11122,.F.);
#14828=ORIENTED_EDGE('',*,*,#11123,.T.);
#14829=ORIENTED_EDGE('',*,*,#11103,.T.);
#14830=ORIENTED_EDGE('',*,*,#11124,.T.);
#14831=ORIENTED_EDGE('',*,*,#11122,.T.);
#14832=ORIENTED_EDGE('',*,*,#11125,.F.);
#14833=ORIENTED_EDGE('',*,*,#11080,.T.);
#14834=ORIENTED_EDGE('',*,*,#11126,.F.);
#14835=ORIENTED_EDGE('',*,*,#11109,.F.);
#14836=ORIENTED_EDGE('',*,*,#11127,.T.);
#14837=ORIENTED_EDGE('',*,*,#10995,.T.);
#14838=ORIENTED_EDGE('',*,*,#10999,.T.);
#14839=ORIENTED_EDGE('',*,*,#11002,.T.);
#14840=ORIENTED_EDGE('',*,*,#11005,.T.);
#14841=ORIENTED_EDGE('',*,*,#11008,.T.);
#14842=ORIENTED_EDGE('',*,*,#11011,.T.);
#14843=ORIENTED_EDGE('',*,*,#11014,.T.);
#14844=ORIENTED_EDGE('',*,*,#11017,.T.);
#14845=ORIENTED_EDGE('',*,*,#11020,.T.);
#14846=ORIENTED_EDGE('',*,*,#11110,.T.);
#14847=ORIENTED_EDGE('',*,*,#11126,.T.);
#14848=ORIENTED_EDGE('',*,*,#11079,.T.);
#14849=ORIENTED_EDGE('',*,*,#11083,.T.);
#14850=ORIENTED_EDGE('',*,*,#11086,.T.);
#14851=ORIENTED_EDGE('',*,*,#11089,.T.);
#14852=ORIENTED_EDGE('',*,*,#11092,.T.);
#14853=ORIENTED_EDGE('',*,*,#11095,.T.);
#14854=ORIENTED_EDGE('',*,*,#11098,.T.);
#14855=ORIENTED_EDGE('',*,*,#11101,.T.);
#14856=ORIENTED_EDGE('',*,*,#11104,.T.);
#14857=ORIENTED_EDGE('',*,*,#11125,.T.);
#14858=ORIENTED_EDGE('',*,*,#11121,.T.);
#14859=ORIENTED_EDGE('',*,*,#11051,.T.);
#14860=ORIENTED_EDGE('',*,*,#11055,.T.);
#14861=ORIENTED_EDGE('',*,*,#11058,.T.);
#14862=ORIENTED_EDGE('',*,*,#11061,.T.);
#14863=ORIENTED_EDGE('',*,*,#11064,.T.);
#14864=ORIENTED_EDGE('',*,*,#11067,.T.);
#14865=ORIENTED_EDGE('',*,*,#11070,.T.);
#14866=ORIENTED_EDGE('',*,*,#11073,.T.);
#14867=ORIENTED_EDGE('',*,*,#11076,.T.);
#14868=ORIENTED_EDGE('',*,*,#11120,.T.);
#14869=ORIENTED_EDGE('',*,*,#11116,.T.);
#14870=ORIENTED_EDGE('',*,*,#11023,.T.);
#14871=ORIENTED_EDGE('',*,*,#11027,.T.);
#14872=ORIENTED_EDGE('',*,*,#11030,.T.);
#14873=ORIENTED_EDGE('',*,*,#11033,.T.);
#14874=ORIENTED_EDGE('',*,*,#11036,.T.);
#14875=ORIENTED_EDGE('',*,*,#11039,.T.);
#14876=ORIENTED_EDGE('',*,*,#11042,.T.);
#14877=ORIENTED_EDGE('',*,*,#11045,.T.);
#14878=ORIENTED_EDGE('',*,*,#11048,.T.);
#14879=ORIENTED_EDGE('',*,*,#11115,.T.);
#14880=ORIENTED_EDGE('',*,*,#11111,.T.);
#14881=ORIENTED_EDGE('',*,*,#11107,.T.);
#14882=ORIENTED_EDGE('',*,*,#10993,.T.);
#14883=ORIENTED_EDGE('',*,*,#11113,.F.);
#14884=ORIENTED_EDGE('',*,*,#11114,.F.);
#14885=ORIENTED_EDGE('',*,*,#11046,.T.);
#14886=ORIENTED_EDGE('',*,*,#11043,.T.);
#14887=ORIENTED_EDGE('',*,*,#11040,.T.);
#14888=ORIENTED_EDGE('',*,*,#11037,.T.);
#14889=ORIENTED_EDGE('',*,*,#11034,.T.);
#14890=ORIENTED_EDGE('',*,*,#11031,.T.);
#14891=ORIENTED_EDGE('',*,*,#11028,.T.);
#14892=ORIENTED_EDGE('',*,*,#11025,.T.);
#14893=ORIENTED_EDGE('',*,*,#11021,.T.);
#14894=ORIENTED_EDGE('',*,*,#11118,.F.);
#14895=ORIENTED_EDGE('',*,*,#11119,.F.);
#14896=ORIENTED_EDGE('',*,*,#11074,.T.);
#14897=ORIENTED_EDGE('',*,*,#11071,.T.);
#14898=ORIENTED_EDGE('',*,*,#11068,.T.);
#14899=ORIENTED_EDGE('',*,*,#11065,.T.);
#14900=ORIENTED_EDGE('',*,*,#11062,.T.);
#14901=ORIENTED_EDGE('',*,*,#11059,.T.);
#14902=ORIENTED_EDGE('',*,*,#11056,.T.);
#14903=ORIENTED_EDGE('',*,*,#11053,.T.);
#14904=ORIENTED_EDGE('',*,*,#11049,.T.);
#14905=ORIENTED_EDGE('',*,*,#11123,.F.);
#14906=ORIENTED_EDGE('',*,*,#11124,.F.);
#14907=ORIENTED_EDGE('',*,*,#11102,.T.);
#14908=ORIENTED_EDGE('',*,*,#11099,.T.);
#14909=ORIENTED_EDGE('',*,*,#11096,.T.);
#14910=ORIENTED_EDGE('',*,*,#11093,.T.);
#14911=ORIENTED_EDGE('',*,*,#11090,.T.);
#14912=ORIENTED_EDGE('',*,*,#11087,.T.);
#14913=ORIENTED_EDGE('',*,*,#11084,.T.);
#14914=ORIENTED_EDGE('',*,*,#11081,.T.);
#14915=ORIENTED_EDGE('',*,*,#11077,.T.);
#14916=ORIENTED_EDGE('',*,*,#11127,.F.);
#14917=ORIENTED_EDGE('',*,*,#11108,.F.);
#14918=ORIENTED_EDGE('',*,*,#11018,.T.);
#14919=ORIENTED_EDGE('',*,*,#11015,.T.);
#14920=ORIENTED_EDGE('',*,*,#11012,.T.);
#14921=ORIENTED_EDGE('',*,*,#11009,.T.);
#14922=ORIENTED_EDGE('',*,*,#11006,.T.);
#14923=ORIENTED_EDGE('',*,*,#11003,.T.);
#14924=ORIENTED_EDGE('',*,*,#11000,.T.);
#14925=ORIENTED_EDGE('',*,*,#10997,.T.);
#14926=ORIENTED_EDGE('',*,*,#11105,.T.);
#17256=CYLINDRICAL_SURFACE('',#20343,0.21);
#18053=ADVANCED_FACE('',(#2729),#1944,.F.);
#18054=ADVANCED_FACE('',(#2730),#1945,.F.);
#18055=ADVANCED_FACE('',(#2731),#1946,.F.);
#18056=ADVANCED_FACE('',(#2732),#1947,.F.);
#18057=ADVANCED_FACE('',(#2733),#1948,.F.);
#18058=ADVANCED_FACE('',(#2734),#1949,.F.);
#18059=ADVANCED_FACE('',(#2735),#1950,.F.);
#18060=ADVANCED_FACE('',(#2736),#1951,.F.);
#18061=ADVANCED_FACE('',(#2737),#1952,.F.);
#18062=ADVANCED_FACE('',(#2738),#1953,.F.);
#18063=ADVANCED_FACE('',(#2739),#1954,.F.);
#18064=ADVANCED_FACE('',(#2740),#1955,.F.);
#18065=ADVANCED_FACE('',(#2741),#1956,.F.);
#18066=ADVANCED_FACE('',(#2742),#1957,.F.);
#18067=ADVANCED_FACE('',(#2743),#1958,.F.);
#18068=ADVANCED_FACE('',(#2744),#1959,.F.);
#18069=ADVANCED_FACE('',(#2745),#1960,.F.);
#18070=ADVANCED_FACE('',(#2746),#1961,.F.);
#18071=ADVANCED_FACE('',(#2747),#1962,.F.);
#18072=ADVANCED_FACE('',(#2748),#1963,.F.);
#18073=ADVANCED_FACE('',(#2749),#1964,.F.);
#18074=ADVANCED_FACE('',(#2750),#1965,.F.);
#18075=ADVANCED_FACE('',(#2751),#1966,.F.);
#18076=ADVANCED_FACE('',(#2752),#1967,.F.);
#18077=ADVANCED_FACE('',(#2753),#1968,.F.);
#18078=ADVANCED_FACE('',(#2754),#1969,.F.);
#18079=ADVANCED_FACE('',(#2755),#1970,.F.);
#18080=ADVANCED_FACE('',(#2756),#1971,.F.);
#18081=ADVANCED_FACE('',(#2757),#1972,.F.);
#18082=ADVANCED_FACE('',(#2758),#1973,.F.);
#18083=ADVANCED_FACE('',(#2759),#1974,.F.);
#18084=ADVANCED_FACE('',(#2760),#1975,.F.);
#18085=ADVANCED_FACE('',(#2761),#1976,.F.);
#18086=ADVANCED_FACE('',(#2762),#1977,.F.);
#18087=ADVANCED_FACE('',(#2763),#1978,.F.);
#18088=ADVANCED_FACE('',(#2764),#1979,.F.);
#18089=ADVANCED_FACE('',(#2765),#17256,.F.);
#18090=ADVANCED_FACE('',(#2766),#1980,.T.);
#18091=ADVANCED_FACE('',(#2767),#1981,.T.);
#18092=ADVANCED_FACE('',(#2768),#1982,.T.);
#18093=ADVANCED_FACE('',(#2769),#1983,.T.);
#18094=ADVANCED_FACE('',(#2770),#1984,.T.);
#18095=ADVANCED_FACE('',(#2771),#1985,.T.);
#18096=ADVANCED_FACE('',(#2772),#1986,.T.);
#18097=ADVANCED_FACE('',(#2773),#1987,.T.);
#18098=ADVANCED_FACE('',(#2774,#1471),#1988,.T.);
#18099=ADVANCED_FACE('',(#2775,#1472),#1989,.F.);
#18594=CLOSED_SHELL('',(#18053,#18054,#18055,#18056,#18057,#18058,#18059,
#18060,#18061,#18062,#18063,#18064,#18065,#18066,#18067,#18068,#18069,#18070,
#18071,#18072,#18073,#18074,#18075,#18076,#18077,#18078,#18079,#18080,#18081,
#18082,#18083,#18084,#18085,#18086,#18087,#18088,#18089,#18090,#18091,#18092,
#18093,#18094,#18095,#18096,#18097,#18098,#18099));
#20306=AXIS2_PLACEMENT_3D('',#29739,#24014,#24015);
#20307=AXIS2_PLACEMENT_3D('',#29740,#24016,#24017);
#20308=AXIS2_PLACEMENT_3D('',#29749,#24022,#24023);
#20309=AXIS2_PLACEMENT_3D('',#29755,#24027,#24028);
#20310=AXIS2_PLACEMENT_3D('',#29761,#24032,#24033);
#20311=AXIS2_PLACEMENT_3D('',#29767,#24037,#24038);
#20312=AXIS2_PLACEMENT_3D('',#29773,#24042,#24043);
#20313=AXIS2_PLACEMENT_3D('',#29779,#24047,#24048);
#20314=AXIS2_PLACEMENT_3D('',#29785,#24052,#24053);
#20315=AXIS2_PLACEMENT_3D('',#29791,#24057,#24058);
#20316=AXIS2_PLACEMENT_3D('',#29797,#24062,#24063);
#20317=AXIS2_PLACEMENT_3D('',#29806,#24068,#24069);
#20318=AXIS2_PLACEMENT_3D('',#29812,#24073,#24074);
#20319=AXIS2_PLACEMENT_3D('',#29818,#24078,#24079);
#20320=AXIS2_PLACEMENT_3D('',#29824,#24083,#24084);
#20321=AXIS2_PLACEMENT_3D('',#29830,#24088,#24089);
#20322=AXIS2_PLACEMENT_3D('',#29836,#24093,#24094);
#20323=AXIS2_PLACEMENT_3D('',#29842,#24098,#24099);
#20324=AXIS2_PLACEMENT_3D('',#29848,#24103,#24104);
#20325=AXIS2_PLACEMENT_3D('',#29854,#24108,#24109);
#20326=AXIS2_PLACEMENT_3D('',#29863,#24114,#24115);
#20327=AXIS2_PLACEMENT_3D('',#29869,#24119,#24120);
#20328=AXIS2_PLACEMENT_3D('',#29875,#24124,#24125);
#20329=AXIS2_PLACEMENT_3D('',#29881,#24129,#24130);
#20330=AXIS2_PLACEMENT_3D('',#29887,#24134,#24135);
#20331=AXIS2_PLACEMENT_3D('',#29893,#24139,#24140);
#20332=AXIS2_PLACEMENT_3D('',#29899,#24144,#24145);
#20333=AXIS2_PLACEMENT_3D('',#29905,#24149,#24150);
#20334=AXIS2_PLACEMENT_3D('',#29911,#24154,#24155);
#20335=AXIS2_PLACEMENT_3D('',#29920,#24160,#24161);
#20336=AXIS2_PLACEMENT_3D('',#29926,#24165,#24166);
#20337=AXIS2_PLACEMENT_3D('',#29932,#24170,#24171);
#20338=AXIS2_PLACEMENT_3D('',#29938,#24175,#24176);
#20339=AXIS2_PLACEMENT_3D('',#29944,#24180,#24181);
#20340=AXIS2_PLACEMENT_3D('',#29950,#24185,#24186);
#20341=AXIS2_PLACEMENT_3D('',#29956,#24190,#24191);
#20342=AXIS2_PLACEMENT_3D('',#29962,#24195,#24196);
#20343=AXIS2_PLACEMENT_3D('',#29968,#24200,#24201);
#20344=AXIS2_PLACEMENT_3D('',#29970,#24202,#24203);
#20345=AXIS2_PLACEMENT_3D('',#29973,#24205,#24206);
#20346=AXIS2_PLACEMENT_3D('',#29974,#24207,#24208);
#20347=AXIS2_PLACEMENT_3D('',#29980,#24212,#24213);
#20348=AXIS2_PLACEMENT_3D('',#29986,#24217,#24218);
#20349=AXIS2_PLACEMENT_3D('',#29989,#24221,#24222);
#20350=AXIS2_PLACEMENT_3D('',#29995,#24226,#24227);
#20351=AXIS2_PLACEMENT_3D('',#29998,#24230,#24231);
#20352=AXIS2_PLACEMENT_3D('',#30004,#24235,#24236);
#20353=AXIS2_PLACEMENT_3D('',#30007,#24239,#24240);
#20354=AXIS2_PLACEMENT_3D('',#30010,#24243,#24244);
#20355=AXIS2_PLACEMENT_3D('',#30011,#24245,#24246);
#24014=DIRECTION('axis',(0.,0.,1.));
#24015=DIRECTION('refdir',(1.,0.,0.));
#24016=DIRECTION('center_axis',(0.,0.,-1.));
#24017=DIRECTION('ref_axis',(0.,1.,0.));
#24018=DIRECTION('',(0.,1.,0.));
#24019=DIRECTION('',(1.,0.,0.));
#24020=DIRECTION('',(0.,-1.,0.));
#24021=DIRECTION('',(1.,0.,0.));
#24022=DIRECTION('center_axis',(0.,1.,-8.88178419700125E-16));
#24023=DIRECTION('ref_axis',(0.,8.88178419700125E-16,1.));
#24024=DIRECTION('',(0.,8.88178419700125E-16,1.));
#24025=DIRECTION('',(1.,0.,0.));
#24026=DIRECTION('',(0.,-8.88178419700125E-16,-1.));
#24027=DIRECTION('center_axis',(0.,-7.40148683083439E-16,-1.));
#24028=DIRECTION('ref_axis',(0.,1.,-7.40148683083439E-16));
#24029=DIRECTION('',(0.,1.,-7.40148683083439E-16));
#24030=DIRECTION('',(1.,0.,0.));
#24031=DIRECTION('',(0.,-1.,7.40148683083439E-16));
#24032=DIRECTION('center_axis',(0.,-0.707106781186547,-0.707106781186548));
#24033=DIRECTION('ref_axis',(0.,0.707106781186548,-0.707106781186547));
#24034=DIRECTION('',(0.,0.707106781186548,-0.707106781186547));
#24035=DIRECTION('',(1.,0.,0.));
#24036=DIRECTION('',(0.,-0.707106781186548,0.707106781186547));
#24037=DIRECTION('center_axis',(0.,-1.,2.77555756156289E-16));
#24038=DIRECTION('ref_axis',(0.,-2.77555756156289E-16,-1.));
#24039=DIRECTION('',(0.,-2.77555756156289E-16,-1.));
#24040=DIRECTION('',(1.,0.,0.));
#24041=DIRECTION('',(0.,2.77555756156289E-16,1.));
#24042=DIRECTION('center_axis',(0.,-0.707106781186547,0.707106781186548));
#24043=DIRECTION('ref_axis',(0.,-0.707106781186548,-0.707106781186547));
#24044=DIRECTION('',(0.,-0.707106781186548,-0.707106781186547));
#24045=DIRECTION('',(1.,0.,0.));
#24046=DIRECTION('',(0.,0.707106781186548,0.707106781186547));
#24047=DIRECTION('center_axis',(0.,7.40148683083438E-16,1.));
#24048=DIRECTION('ref_axis',(0.,-1.,7.40148683083438E-16));
#24049=DIRECTION('',(0.,-1.,7.40148683083438E-16));
#24050=DIRECTION('',(1.,0.,0.));
#24051=DIRECTION('',(0.,1.,-7.40148683083438E-16));
#24052=DIRECTION('center_axis',(0.,1.,-4.44089209850063E-16));
#24053=DIRECTION('ref_axis',(0.,4.44089209850063E-16,1.));
#24054=DIRECTION('',(0.,4.44089209850063E-16,1.));
#24055=DIRECTION('',(1.,0.,0.));
#24056=DIRECTION('',(0.,-4.44089209850063E-16,-1.));
#24057=DIRECTION('center_axis',(0.,2.41352831440251E-16,1.));
#24058=DIRECTION('ref_axis',(0.,-1.,2.41352831440251E-16));
#24059=DIRECTION('',(0.,-1.,2.41352831440251E-16));
#24060=DIRECTION('',(-1.,0.,0.));
#24061=DIRECTION('',(0.,1.,-2.41352831440251E-16));
#24062=DIRECTION('center_axis',(0.,-1.,2.41352831440251E-16));
#24063=DIRECTION('ref_axis',(0.,-2.41352831440251E-16,-1.));
#24064=DIRECTION('',(0.,-2.41352831440251E-16,-1.));
#24065=DIRECTION('',(1.,0.,0.));
#24066=DIRECTION('',(0.,2.41352831440251E-16,1.));
#24067=DIRECTION('',(1.,0.,0.));
#24068=DIRECTION('center_axis',(0.,0.,-1.));
#24069=DIRECTION('ref_axis',(0.,1.,0.));
#24070=DIRECTION('',(0.,1.,0.));
#24071=DIRECTION('',(1.,0.,0.));
#24072=DIRECTION('',(0.,-1.,0.));
#24073=DIRECTION('center_axis',(0.,-1.,0.));
#24074=DIRECTION('ref_axis',(0.,0.,-1.));
#24075=DIRECTION('',(0.,0.,-1.));
#24076=DIRECTION('',(1.,0.,0.));
#24077=DIRECTION('',(0.,0.,1.));
#24078=DIRECTION('center_axis',(0.,-0.707106781186547,0.707106781186548));
#24079=DIRECTION('ref_axis',(0.,-0.707106781186548,-0.707106781186547));
#24080=DIRECTION('',(0.,-0.707106781186548,-0.707106781186547));
#24081=DIRECTION('',(1.,0.,0.));
#24082=DIRECTION('',(0.,0.707106781186548,0.707106781186547));
#24083=DIRECTION('center_axis',(0.,0.,1.));
#24084=DIRECTION('ref_axis',(0.,-1.,0.));
#24085=DIRECTION('',(0.,-1.,0.));
#24086=DIRECTION('',(1.,0.,0.));
#24087=DIRECTION('',(0.,1.,0.));
#24088=DIRECTION('center_axis',(0.,0.707106781186548,0.707106781186547));
#24089=DIRECTION('ref_axis',(0.,-0.707106781186547,0.707106781186548));
#24090=DIRECTION('',(0.,-0.707106781186547,0.707106781186548));
#24091=DIRECTION('',(1.,0.,0.));
#24092=DIRECTION('',(0.,0.707106781186547,-0.707106781186548));
#24093=DIRECTION('center_axis',(0.,1.,0.));
#24094=DIRECTION('ref_axis',(0.,0.,1.));
#24095=DIRECTION('',(0.,0.,1.));
#24096=DIRECTION('',(1.,0.,0.));
#24097=DIRECTION('',(0.,0.,-1.));
#24098=DIRECTION('center_axis',(0.,0.,-1.));
#24099=DIRECTION('ref_axis',(0.,1.,0.));
#24100=DIRECTION('',(0.,1.,0.));
#24101=DIRECTION('',(1.,0.,0.));
#24102=DIRECTION('',(0.,-1.,0.));
#24103=DIRECTION('center_axis',(0.,1.,-2.41352831440251E-16));
#24104=DIRECTION('ref_axis',(0.,2.41352831440251E-16,1.));
#24105=DIRECTION('',(0.,2.41352831440251E-16,1.));
#24106=DIRECTION('',(-1.,0.,0.));
#24107=DIRECTION('',(0.,-2.41352831440251E-16,-1.));
#24108=DIRECTION('center_axis',(0.,0.,1.));
#24109=DIRECTION('ref_axis',(0.,-1.,0.));
#24110=DIRECTION('',(0.,-1.,0.));
#24111=DIRECTION('',(1.,0.,0.));
#24112=DIRECTION('',(0.,1.,0.));
#24113=DIRECTION('',(1.,0.,0.));
#24114=DIRECTION('center_axis',(0.,-1.,0.));
#24115=DIRECTION('ref_axis',(0.,0.,-1.));
#24116=DIRECTION('',(0.,0.,-1.));
#24117=DIRECTION('',(1.,0.,0.));
#24118=DIRECTION('',(0.,0.,1.));
#24119=DIRECTION('center_axis',(0.,0.,1.));
#24120=DIRECTION('ref_axis',(0.,-1.,0.));
#24121=DIRECTION('',(0.,-1.,0.));
#24122=DIRECTION('',(1.,0.,0.));
#24123=DIRECTION('',(0.,1.,0.));
#24124=DIRECTION('center_axis',(0.,0.707106781186548,0.707106781186548));
#24125=DIRECTION('ref_axis',(0.,-0.707106781186548,0.707106781186548));
#24126=DIRECTION('',(0.,-0.707106781186548,0.707106781186548));
#24127=DIRECTION('',(1.,0.,0.));
#24128=DIRECTION('',(0.,0.707106781186548,-0.707106781186548));
#24129=DIRECTION('center_axis',(0.,1.,0.));
#24130=DIRECTION('ref_axis',(0.,0.,1.));
#24131=DIRECTION('',(0.,0.,1.));
#24132=DIRECTION('',(1.,0.,0.));
#24133=DIRECTION('',(0.,0.,-1.));
#24134=DIRECTION('center_axis',(0.,0.707106781186548,-0.707106781186547));
#24135=DIRECTION('ref_axis',(0.,0.707106781186547,0.707106781186548));
#24136=DIRECTION('',(0.,0.707106781186547,0.707106781186548));
#24137=DIRECTION('',(1.,0.,0.));
#24138=DIRECTION('',(0.,-0.707106781186547,-0.707106781186548));
#24139=DIRECTION('center_axis',(0.,-7.40148683083438E-16,-1.));
#24140=DIRECTION('ref_axis',(0.,1.,-7.40148683083438E-16));
#24141=DIRECTION('',(0.,1.,-7.40148683083438E-16));
#24142=DIRECTION('',(1.,0.,0.));
#24143=DIRECTION('',(0.,-1.,7.40148683083438E-16));
#24144=DIRECTION('center_axis',(0.,-1.,0.));
#24145=DIRECTION('ref_axis',(0.,0.,-1.));
#24146=DIRECTION('',(0.,0.,-1.));
#24147=DIRECTION('',(1.,0.,0.));
#24148=DIRECTION('',(0.,0.,1.));
#24149=DIRECTION('center_axis',(0.,0.,-1.));
#24150=DIRECTION('ref_axis',(0.,1.,0.));
#24151=DIRECTION('',(0.,1.,0.));
#24152=DIRECTION('',(-1.,0.,0.));
#24153=DIRECTION('',(0.,-1.,0.));
#24154=DIRECTION('center_axis',(0.,1.,0.));
#24155=DIRECTION('ref_axis',(0.,0.,1.));
#24156=DIRECTION('',(0.,0.,1.));
#24157=DIRECTION('',(1.,0.,0.));
#24158=DIRECTION('',(0.,0.,-1.));
#24159=DIRECTION('',(1.,0.,0.));
#24160=DIRECTION('center_axis',(0.,0.,1.));
#24161=DIRECTION('ref_axis',(0.,-1.,0.));
#24162=DIRECTION('',(0.,-1.,0.));
#24163=DIRECTION('',(1.,0.,0.));
#24164=DIRECTION('',(0.,1.,0.));
#24165=DIRECTION('center_axis',(0.,1.,0.));
#24166=DIRECTION('ref_axis',(0.,0.,1.));
#24167=DIRECTION('',(0.,0.,1.));
#24168=DIRECTION('',(1.,0.,0.));
#24169=DIRECTION('',(0.,0.,-1.));
#24170=DIRECTION('center_axis',(0.,0.707106781186547,-0.707106781186548));
#24171=DIRECTION('ref_axis',(0.,0.707106781186548,0.707106781186547));
#24172=DIRECTION('',(0.,0.707106781186548,0.707106781186547));
#24173=DIRECTION('',(1.,0.,0.));
#24174=DIRECTION('',(0.,-0.707106781186548,-0.707106781186547));
#24175=DIRECTION('center_axis',(0.,0.,-1.));
#24176=DIRECTION('ref_axis',(0.,1.,0.));
#24177=DIRECTION('',(0.,1.,0.));
#24178=DIRECTION('',(1.,0.,0.));
#24179=DIRECTION('',(0.,-1.,0.));
#24180=DIRECTION('center_axis',(0.,-0.707106781186547,-0.707106781186548));
#24181=DIRECTION('ref_axis',(0.,0.707106781186548,-0.707106781186547));
#24182=DIRECTION('',(0.,0.707106781186548,-0.707106781186547));
#24183=DIRECTION('',(1.,0.,0.));
#24184=DIRECTION('',(0.,-0.707106781186548,0.707106781186547));
#24185=DIRECTION('center_axis',(0.,-1.,0.));
#24186=DIRECTION('ref_axis',(0.,0.,-1.));
#24187=DIRECTION('',(0.,0.,-1.));
#24188=DIRECTION('',(1.,0.,0.));
#24189=DIRECTION('',(0.,0.,1.));
#24190=DIRECTION('center_axis',(0.,0.,1.));
#24191=DIRECTION('ref_axis',(0.,-1.,0.));
#24192=DIRECTION('',(0.,-1.,0.));
#24193=DIRECTION('',(1.,0.,0.));
#24194=DIRECTION('',(0.,1.,0.));
#24195=DIRECTION('center_axis',(0.,-1.,0.));
#24196=DIRECTION('ref_axis',(0.,0.,-1.));
#24197=DIRECTION('',(0.,0.,-1.));
#24198=DIRECTION('',(-1.,0.,0.));
#24199=DIRECTION('',(0.,0.,1.));
#24200=DIRECTION('center_axis',(1.,0.,0.));
#24201=DIRECTION('ref_axis',(0.,0.,-1.));
#24202=DIRECTION('center_axis',(1.,0.,0.));
#24203=DIRECTION('ref_axis',(0.,0.,-1.));
#24204=DIRECTION('',(1.,0.,0.));
#24205=DIRECTION('center_axis',(-1.,0.,0.));
#24206=DIRECTION('ref_axis',(0.,0.,-1.));
#24207=DIRECTION('center_axis',(0.,1.,0.));
#24208=DIRECTION('ref_axis',(0.,0.,1.));
#24209=DIRECTION('',(0.,0.,1.));
#24210=DIRECTION('',(1.,0.,0.));
#24211=DIRECTION('',(0.,0.,1.));
#24212=DIRECTION('center_axis',(0.,1.,0.));
#24213=DIRECTION('ref_axis',(0.,0.,1.));
#24214=DIRECTION('',(0.,0.,1.));
#24215=DIRECTION('',(1.,0.,0.));
#24216=DIRECTION('',(0.,0.,1.));
#24217=DIRECTION('center_axis',(0.,0.,-1.));
#24218=DIRECTION('ref_axis',(0.,1.,0.));
#24219=DIRECTION('',(0.,1.,0.));
#24220=DIRECTION('',(0.,1.,0.));
#24221=DIRECTION('center_axis',(0.,0.,-1.));
#24222=DIRECTION('ref_axis',(0.,1.,0.));
#24223=DIRECTION('',(0.,1.,0.));
#24224=DIRECTION('',(1.,0.,0.));
#24225=DIRECTION('',(0.,1.,0.));
#24226=DIRECTION('center_axis',(0.,-1.,0.));
#24227=DIRECTION('ref_axis',(0.,0.,-1.));
#24228=DIRECTION('',(0.,0.,-1.));
#24229=DIRECTION('',(0.,0.,-1.));
#24230=DIRECTION('center_axis',(0.,-1.,0.));
#24231=DIRECTION('ref_axis',(0.,0.,-1.));
#24232=DIRECTION('',(0.,0.,-1.));
#24233=DIRECTION('',(1.,0.,0.));
#24234=DIRECTION('',(0.,0.,-1.));
#24235=DIRECTION('center_axis',(0.,0.,1.));
#24236=DIRECTION('ref_axis',(0.,-1.,0.));
#24237=DIRECTION('',(0.,-1.,0.));
#24238=DIRECTION('',(0.,-1.,0.));
#24239=DIRECTION('center_axis',(0.,0.,1.));
#24240=DIRECTION('ref_axis',(0.,-1.,0.));
#24241=DIRECTION('',(0.,-1.,0.));
#24242=DIRECTION('',(0.,-1.,0.));
#24243=DIRECTION('center_axis',(1.,0.,0.));
#24244=DIRECTION('ref_axis',(0.,0.,-1.));
#24245=DIRECTION('center_axis',(1.,0.,0.));
#24246=DIRECTION('ref_axis',(0.,0.,-1.));
#29739=CARTESIAN_POINT('',(0.,0.,0.));
#29740=CARTESIAN_POINT('Origin',(-0.1,0.82,-0.3));
#29741=CARTESIAN_POINT('',(0.,0.82,-0.3));
#29742=CARTESIAN_POINT('',(0.,1.,-0.3));
#29743=CARTESIAN_POINT('',(0.,0.41,-0.3));
#29744=CARTESIAN_POINT('',(40.,0.82,-0.3));
#29745=CARTESIAN_POINT('',(-0.1,0.82,-0.3));
#29746=CARTESIAN_POINT('',(40.,1.,-0.3));
#29747=CARTESIAN_POINT('',(40.,0.41,-0.3));
#29748=CARTESIAN_POINT('',(-0.05,1.,-0.3));
#29749=CARTESIAN_POINT('Origin',(-0.1,0.82,-0.55));
#29750=CARTESIAN_POINT('',(0.,0.82,-0.55));
#29751=CARTESIAN_POINT('',(0.,0.82,-0.275));
#29752=CARTESIAN_POINT('',(40.,0.82,-0.55));
#29753=CARTESIAN_POINT('',(-0.1,0.82,-0.55));
#29754=CARTESIAN_POINT('',(40.,0.82,-0.275));
#29755=CARTESIAN_POINT('Origin',(-0.1,0.67,-0.55));
#29756=CARTESIAN_POINT('',(0.,0.67,-0.55));
#29757=CARTESIAN_POINT('',(0.,0.335,-0.55));
#29758=CARTESIAN_POINT('',(40.,0.67,-0.55));
#29759=CARTESIAN_POINT('',(-0.1,0.67,-0.55));
#29760=CARTESIAN_POINT('',(40.,0.335,-0.55));
#29761=CARTESIAN_POINT('Origin',(-0.1,0.42,-0.3));
#29762=CARTESIAN_POINT('',(0.,0.42,-0.3));
#29763=CARTESIAN_POINT('',(0.,0.24,-0.12));
#29764=CARTESIAN_POINT('',(40.,0.42,-0.3));
#29765=CARTESIAN_POINT('',(-0.1,0.42,-0.3));
#29766=CARTESIAN_POINT('',(40.,0.24,-0.12));
#29767=CARTESIAN_POINT('Origin',(-0.1,0.42,0.3));
#29768=CARTESIAN_POINT('',(0.,0.42,0.3));
#29769=CARTESIAN_POINT('',(0.,0.42,0.15));
#29770=CARTESIAN_POINT('',(40.,0.42,0.3));
#29771=CARTESIAN_POINT('',(-0.1,0.42,0.3));
#29772=CARTESIAN_POINT('',(40.,0.42,0.15));
#29773=CARTESIAN_POINT('Origin',(-0.1,0.67,0.55));
#29774=CARTESIAN_POINT('',(0.,0.67,0.55));
#29775=CARTESIAN_POINT('',(6.93889390390723E-18,0.365,0.245));
#29776=CARTESIAN_POINT('',(40.,0.67,0.55));
#29777=CARTESIAN_POINT('',(-0.1,0.67,0.55));
#29778=CARTESIAN_POINT('',(40.,0.365,0.245));
#29779=CARTESIAN_POINT('Origin',(-0.1,0.82,0.55));
#29780=CARTESIAN_POINT('',(0.,0.82,0.55));
#29781=CARTESIAN_POINT('',(0.,0.41,0.55));
#29782=CARTESIAN_POINT('',(40.,0.82,0.55));
#29783=CARTESIAN_POINT('',(-0.1,0.82,0.55));
#29784=CARTESIAN_POINT('',(40.,0.41,0.55));
#29785=CARTESIAN_POINT('Origin',(-0.1,0.82,0.3));
#29786=CARTESIAN_POINT('',(0.,0.82,0.3));
#29787=CARTESIAN_POINT('',(0.,0.82,0.15));
#29788=CARTESIAN_POINT('',(40.,0.82,0.3));
#29789=CARTESIAN_POINT('',(-0.1,0.82,0.3));
#29790=CARTESIAN_POINT('',(40.,0.82,0.15));
#29791=CARTESIAN_POINT('Origin',(-0.1,1.05,0.3));
#29792=CARTESIAN_POINT('',(0.,1.,0.3));
#29793=CARTESIAN_POINT('',(0.,0.525,0.3));
#29794=CARTESIAN_POINT('',(40.,1.,0.3));
#29795=CARTESIAN_POINT('',(-0.05,1.,0.3));
#29796=CARTESIAN_POINT('',(40.,0.525,0.3));
#29797=CARTESIAN_POINT('Origin',(-0.1,-0.3,-0.82));
#29798=CARTESIAN_POINT('',(0.,-0.3,-0.82));
#29799=CARTESIAN_POINT('',(0.,-0.3,-1.));
#29800=CARTESIAN_POINT('',(0.,-0.3,-0.41));
#29801=CARTESIAN_POINT('',(40.,-0.3,-0.82));
#29802=CARTESIAN_POINT('',(-0.1,-0.3,-0.82));
#29803=CARTESIAN_POINT('',(40.,-0.3,-1.));
#29804=CARTESIAN_POINT('',(40.,-0.3,-0.41));
#29805=CARTESIAN_POINT('',(-0.05,-0.3,-1.));
#29806=CARTESIAN_POINT('Origin',(-0.1,-0.55,-0.82));
#29807=CARTESIAN_POINT('',(0.,-0.55,-0.82));
#29808=CARTESIAN_POINT('',(0.,-0.275,-0.82));
#29809=CARTESIAN_POINT('',(40.,-0.55,-0.82));
#29810=CARTESIAN_POINT('',(-0.1,-0.55,-0.82));
#29811=CARTESIAN_POINT('',(40.,-0.275,-0.82));
#29812=CARTESIAN_POINT('Origin',(-0.1,-0.55,-0.67));
#29813=CARTESIAN_POINT('',(0.,-0.55,-0.67));
#29814=CARTESIAN_POINT('',(0.,-0.55,-0.335));
#29815=CARTESIAN_POINT('',(40.,-0.55,-0.67));
#29816=CARTESIAN_POINT('',(-0.1,-0.55,-0.67));
#29817=CARTESIAN_POINT('',(40.,-0.55,-0.335));
#29818=CARTESIAN_POINT('Origin',(-0.1,-0.3,-0.42));
#29819=CARTESIAN_POINT('',(0.,-0.3,-0.42));
#29820=CARTESIAN_POINT('',(0.,-0.12,-0.24));
#29821=CARTESIAN_POINT('',(40.,-0.3,-0.42));
#29822=CARTESIAN_POINT('',(-0.1,-0.3,-0.42));
#29823=CARTESIAN_POINT('',(40.,-0.12,-0.24));
#29824=CARTESIAN_POINT('Origin',(-0.1,0.3,-0.42));
#29825=CARTESIAN_POINT('',(0.,0.3,-0.42));
#29826=CARTESIAN_POINT('',(0.,0.15,-0.42));
#29827=CARTESIAN_POINT('',(40.,0.3,-0.42));
#29828=CARTESIAN_POINT('',(-0.1,0.3,-0.42));
#29829=CARTESIAN_POINT('',(40.,0.15,-0.42));
#29830=CARTESIAN_POINT('Origin',(-0.1,0.55,-0.67));
#29831=CARTESIAN_POINT('',(0.,0.55,-0.67));
#29832=CARTESIAN_POINT('',(0.,0.245,-0.365));
#29833=CARTESIAN_POINT('',(40.,0.55,-0.67));
#29834=CARTESIAN_POINT('',(-0.1,0.55,-0.67));
#29835=CARTESIAN_POINT('',(40.,0.245,-0.365));
#29836=CARTESIAN_POINT('Origin',(-0.1,0.55,-0.82));
#29837=CARTESIAN_POINT('',(0.,0.55,-0.82));
#29838=CARTESIAN_POINT('',(0.,0.55,-0.41));
#29839=CARTESIAN_POINT('',(40.,0.55,-0.82));
#29840=CARTESIAN_POINT('',(-0.1,0.55,-0.82));
#29841=CARTESIAN_POINT('',(40.,0.55,-0.41));
#29842=CARTESIAN_POINT('Origin',(-0.1,0.3,-0.82));
#29843=CARTESIAN_POINT('',(0.,0.3,-0.82));
#29844=CARTESIAN_POINT('',(0.,0.15,-0.82));
#29845=CARTESIAN_POINT('',(40.,0.3,-0.82));
#29846=CARTESIAN_POINT('',(-0.1,0.3,-0.82));
#29847=CARTESIAN_POINT('',(40.,0.15,-0.82));
#29848=CARTESIAN_POINT('Origin',(-0.1,0.3,-1.05));
#29849=CARTESIAN_POINT('',(0.,0.3,-1.));
#29850=CARTESIAN_POINT('',(0.,0.3,-0.525));
#29851=CARTESIAN_POINT('',(40.,0.3,-1.));
#29852=CARTESIAN_POINT('',(-0.05,0.3,-1.));
#29853=CARTESIAN_POINT('',(40.,0.3,-0.525));
#29854=CARTESIAN_POINT('Origin',(-0.1,-0.82,0.3));
#29855=CARTESIAN_POINT('',(0.,-0.82,0.3));
#29856=CARTESIAN_POINT('',(0.,-1.,0.3));
#29857=CARTESIAN_POINT('',(0.,-0.41,0.3));
#29858=CARTESIAN_POINT('',(40.,-0.82,0.3));
#29859=CARTESIAN_POINT('',(-0.1,-0.82,0.3));
#29860=CARTESIAN_POINT('',(40.,-1.,0.3));
#29861=CARTESIAN_POINT('',(40.,-0.41,0.3));
#29862=CARTESIAN_POINT('',(-0.05,-1.,0.3));
#29863=CARTESIAN_POINT('Origin',(-0.1,-0.82,0.55));
#29864=CARTESIAN_POINT('',(0.,-0.82,0.55));
#29865=CARTESIAN_POINT('',(0.,-0.82,0.275));
#29866=CARTESIAN_POINT('',(40.,-0.82,0.55));
#29867=CARTESIAN_POINT('',(-0.1,-0.82,0.55));
#29868=CARTESIAN_POINT('',(40.,-0.82,0.275));
#29869=CARTESIAN_POINT('Origin',(-0.1,-0.67,0.55));
#29870=CARTESIAN_POINT('',(0.,-0.67,0.55));
#29871=CARTESIAN_POINT('',(0.,-0.335,0.55));
#29872=CARTESIAN_POINT('',(40.,-0.67,0.55));
#29873=CARTESIAN_POINT('',(-0.1,-0.67,0.55));
#29874=CARTESIAN_POINT('',(40.,-0.335,0.55));
#29875=CARTESIAN_POINT('Origin',(-0.1,-0.42,0.3));
#29876=CARTESIAN_POINT('',(0.,-0.42,0.3));
#29877=CARTESIAN_POINT('',(-6.93889390390723E-18,-0.24,0.12));
#29878=CARTESIAN_POINT('',(40.,-0.42,0.3));
#29879=CARTESIAN_POINT('',(-0.1,-0.42,0.3));
#29880=CARTESIAN_POINT('',(40.,-0.24,0.12));
#29881=CARTESIAN_POINT('Origin',(-0.1,-0.42,-0.3));
#29882=CARTESIAN_POINT('',(0.,-0.42,-0.3));
#29883=CARTESIAN_POINT('',(0.,-0.42,-0.15));
#29884=CARTESIAN_POINT('',(40.,-0.42,-0.3));
#29885=CARTESIAN_POINT('',(-0.1,-0.42,-0.3));
#29886=CARTESIAN_POINT('',(40.,-0.42,-0.15));
#29887=CARTESIAN_POINT('Origin',(-0.1,-0.67,-0.55));
#29888=CARTESIAN_POINT('',(0.,-0.67,-0.55));
#29889=CARTESIAN_POINT('',(0.,-0.365,-0.245));
#29890=CARTESIAN_POINT('',(40.,-0.67,-0.55));
#29891=CARTESIAN_POINT('',(-0.1,-0.67,-0.55));
#29892=CARTESIAN_POINT('',(40.,-0.365,-0.245));
#29893=CARTESIAN_POINT('Origin',(-0.1,-0.82,-0.55));
#29894=CARTESIAN_POINT('',(0.,-0.82,-0.55));
#29895=CARTESIAN_POINT('',(0.,-0.41,-0.55));
#29896=CARTESIAN_POINT('',(40.,-0.82,-0.55));
#29897=CARTESIAN_POINT('',(-0.1,-0.82,-0.55));
#29898=CARTESIAN_POINT('',(40.,-0.41,-0.55));
#29899=CARTESIAN_POINT('Origin',(-0.1,-0.82,-0.3));
#29900=CARTESIAN_POINT('',(0.,-0.82,-0.3));
#29901=CARTESIAN_POINT('',(0.,-0.82,-0.15));
#29902=CARTESIAN_POINT('',(40.,-0.82,-0.3));
#29903=CARTESIAN_POINT('',(-0.1,-0.82,-0.3));
#29904=CARTESIAN_POINT('',(40.,-0.82,-0.15));
#29905=CARTESIAN_POINT('Origin',(-0.1,-1.05,-0.3));
#29906=CARTESIAN_POINT('',(0.,-1.,-0.3));
#29907=CARTESIAN_POINT('',(0.,-0.525,-0.3));
#29908=CARTESIAN_POINT('',(40.,-1.,-0.3));
#29909=CARTESIAN_POINT('',(-0.05,-1.,-0.3));
#29910=CARTESIAN_POINT('',(40.,-0.525,-0.3));
#29911=CARTESIAN_POINT('Origin',(-0.1,0.3,0.82));
#29912=CARTESIAN_POINT('',(0.,0.3,0.82));
#29913=CARTESIAN_POINT('',(0.,0.3,1.));
#29914=CARTESIAN_POINT('',(0.,0.3,0.41));
#29915=CARTESIAN_POINT('',(40.,0.3,0.82));
#29916=CARTESIAN_POINT('',(-0.1,0.3,0.82));
#29917=CARTESIAN_POINT('',(40.,0.3,1.));
#29918=CARTESIAN_POINT('',(40.,0.3,0.41));
#29919=CARTESIAN_POINT('',(-0.05,0.3,1.));
#29920=CARTESIAN_POINT('Origin',(-0.1,0.55,0.82));
#29921=CARTESIAN_POINT('',(0.,0.55,0.82));
#29922=CARTESIAN_POINT('',(0.,0.275,0.82));
#29923=CARTESIAN_POINT('',(40.,0.55,0.82));
#29924=CARTESIAN_POINT('',(-0.1,0.55,0.82));
#29925=CARTESIAN_POINT('',(40.,0.275,0.82));
#29926=CARTESIAN_POINT('Origin',(-0.1,0.55,0.67));
#29927=CARTESIAN_POINT('',(0.,0.55,0.67));
#29928=CARTESIAN_POINT('',(0.,0.55,0.335));
#29929=CARTESIAN_POINT('',(40.,0.55,0.67));
#29930=CARTESIAN_POINT('',(-0.1,0.55,0.67));
#29931=CARTESIAN_POINT('',(40.,0.55,0.335));
#29932=CARTESIAN_POINT('Origin',(-0.1,0.3,0.42));
#29933=CARTESIAN_POINT('',(0.,0.3,0.42));
#29934=CARTESIAN_POINT('',(6.93889390390723E-18,0.12,0.24));
#29935=CARTESIAN_POINT('',(40.,0.3,0.42));
#29936=CARTESIAN_POINT('',(-0.1,0.3,0.42));
#29937=CARTESIAN_POINT('',(40.,0.12,0.24));
#29938=CARTESIAN_POINT('Origin',(-0.1,-0.3,0.42));
#29939=CARTESIAN_POINT('',(0.,-0.3,0.42));
#29940=CARTESIAN_POINT('',(0.,-0.15,0.42));
#29941=CARTESIAN_POINT('',(40.,-0.3,0.42));
#29942=CARTESIAN_POINT('',(-0.1,-0.3,0.42));
#29943=CARTESIAN_POINT('',(40.,-0.15,0.42));
#29944=CARTESIAN_POINT('Origin',(-0.1,-0.55,0.67));
#29945=CARTESIAN_POINT('',(0.,-0.55,0.67));
#29946=CARTESIAN_POINT('',(6.93889390390723E-18,-0.245,0.365));
#29947=CARTESIAN_POINT('',(40.,-0.55,0.67));
#29948=CARTESIAN_POINT('',(-0.1,-0.55,0.67));
#29949=CARTESIAN_POINT('',(40.,-0.245,0.365));
#29950=CARTESIAN_POINT('Origin',(-0.1,-0.55,0.82));
#29951=CARTESIAN_POINT('',(0.,-0.55,0.82));
#29952=CARTESIAN_POINT('',(0.,-0.55,0.41));
#29953=CARTESIAN_POINT('',(40.,-0.55,0.82));
#29954=CARTESIAN_POINT('',(-0.1,-0.55,0.82));
#29955=CARTESIAN_POINT('',(40.,-0.55,0.41));
#29956=CARTESIAN_POINT('Origin',(-0.1,-0.3,0.82));
#29957=CARTESIAN_POINT('',(0.,-0.3,0.82));
#29958=CARTESIAN_POINT('',(0.,-0.15,0.82));
#29959=CARTESIAN_POINT('',(40.,-0.3,0.82));
#29960=CARTESIAN_POINT('',(-0.1,-0.3,0.82));
#29961=CARTESIAN_POINT('',(40.,-0.15,0.82));
#29962=CARTESIAN_POINT('Origin',(-0.1,-0.3,1.05));
#29963=CARTESIAN_POINT('',(0.,-0.3,1.));
#29964=CARTESIAN_POINT('',(0.,-0.3,0.525));
#29965=CARTESIAN_POINT('',(40.,-0.3,1.));
#29966=CARTESIAN_POINT('',(-0.05,-0.3,1.));
#29967=CARTESIAN_POINT('',(40.,-0.3,0.525));
#29968=CARTESIAN_POINT('Origin',(-0.1,0.,0.));
#29969=CARTESIAN_POINT('',(0.,-2.57175827820944E-17,0.21));
#29970=CARTESIAN_POINT('Origin',(0.,0.,0.));
#29971=CARTESIAN_POINT('',(40.,2.57175827820944E-17,0.21));
#29972=CARTESIAN_POINT('',(-0.1,-2.57175827820944E-17,0.21));
#29973=CARTESIAN_POINT('Origin',(40.,0.,0.));
#29974=CARTESIAN_POINT('Origin',(0.,1.,-1.));
#29975=CARTESIAN_POINT('',(0.,1.,1.));
#29976=CARTESIAN_POINT('',(0.,1.,-1.));
#29977=CARTESIAN_POINT('',(40.,1.,1.));
#29978=CARTESIAN_POINT('',(0.,1.,1.));
#29979=CARTESIAN_POINT('',(40.,1.,-1.));
#29980=CARTESIAN_POINT('Origin',(0.,1.,-1.));
#29981=CARTESIAN_POINT('',(40.,1.,-1.));
#29982=CARTESIAN_POINT('',(40.,1.,-1.));
#29983=CARTESIAN_POINT('',(0.,1.,-1.));
#29984=CARTESIAN_POINT('',(0.,1.,-1.));
#29985=CARTESIAN_POINT('',(0.,1.,-1.));
#29986=CARTESIAN_POINT('Origin',(0.,-1.,-1.));
#29987=CARTESIAN_POINT('',(0.,-1.,-1.));
#29988=CARTESIAN_POINT('',(40.,-1.,-1.));
#29989=CARTESIAN_POINT('Origin',(0.,-1.,-1.));
#29990=CARTESIAN_POINT('',(40.,-1.,-1.));
#29991=CARTESIAN_POINT('',(40.,-1.,-1.));
#29992=CARTESIAN_POINT('',(0.,-1.,-1.));
#29993=CARTESIAN_POINT('',(0.,-1.,-1.));
#29994=CARTESIAN_POINT('',(0.,-1.,-1.));
#29995=CARTESIAN_POINT('Origin',(0.,-1.,1.));
#29996=CARTESIAN_POINT('',(0.,-1.,1.));
#29997=CARTESIAN_POINT('',(40.,-1.,1.));
#29998=CARTESIAN_POINT('Origin',(0.,-1.,1.));
#29999=CARTESIAN_POINT('',(40.,-1.,1.));
#30000=CARTESIAN_POINT('',(40.,-1.,1.));
#30001=CARTESIAN_POINT('',(0.,-1.,1.));
#30002=CARTESIAN_POINT('',(0.,-1.,1.));
#30003=CARTESIAN_POINT('',(0.,-1.,1.));
#30004=CARTESIAN_POINT('Origin',(0.,1.,1.));
#30005=CARTESIAN_POINT('',(0.,1.,1.));
#30006=CARTESIAN_POINT('',(40.,1.,1.));
#30007=CARTESIAN_POINT('Origin',(0.,1.,1.));
#30008=CARTESIAN_POINT('',(40.,1.,1.));
#30009=CARTESIAN_POINT('',(0.,1.,1.));
#30010=CARTESIAN_POINT('Origin',(40.,0.,0.));
#30011=CARTESIAN_POINT('Origin',(0.,0.,0.));
#43425=UNCERTAINTY_MEASURE_WITH_UNIT(LENGTH_MEASURE(0.001),#43522,
'DISTANCE_ACCURACY_VALUE',
'Maximum model space distance between geometric entities at asserted c
onnectivities');
#43453=UNCERTAINTY_MEASURE_WITH_UNIT(LENGTH_MEASURE(0.001),#43522,
'DISTANCE_ACCURACY_VALUE',
'Maximum model space distance between geometric entities at asserted c
onnectivities');
#43493=(
GEOMETRIC_REPRESENTATION_CONTEXT(3)
GLOBAL_UNCERTAINTY_ASSIGNED_CONTEXT((#43425))
GLOBAL_UNIT_ASSIGNED_CONTEXT((#43522,#43524,#43525))
REPRESENTATION_CONTEXT('','3D')
);
#43521=(
GEOMETRIC_REPRESENTATION_CONTEXT(3)
GLOBAL_UNCERTAINTY_ASSIGNED_CONTEXT((#43453))
GLOBAL_UNIT_ASSIGNED_CONTEXT((#43522,#43524,#43525))
REPRESENTATION_CONTEXT('','3D')
);
#43522=(
LENGTH_UNIT()
NAMED_UNIT(*)
SI_UNIT(.CENTI.,.METRE.)
);
#43524=(
NAMED_UNIT(*)
PLANE_ANGLE_UNIT()
SI_UNIT($,.RADIAN.)
);
#43525=(
NAMED_UNIT(*)
SI_UNIT($,.STERADIAN.)
SOLID_ANGLE_UNIT()
);
#43565=SHAPE_DEFINITION_REPRESENTATION(#43642,#43833);
#43642=PRODUCT_DEFINITION_SHAPE('',$,#43901);
#43833=SHAPE_REPRESENTATION('',(#20306),#43493);
#43861=PRODUCT_DEFINITION_CONTEXT('part definition',#44064,'design');
#43901=PRODUCT_DEFINITION('Slotted Extrusion - 20 x 20 x 400 mm',
'Slotted Extrusion - 20 x 20 x 400 mm',#43968,#43861);
#43968=PRODUCT_DEFINITION_FORMATION('',$,#44105);
#44064=APPLICATION_CONTEXT(
'Core Data for Automotive Mechanical Design Process');
#44065=PRODUCT_CONTEXT('part definition',#44064,'mechanical');
#44105=PRODUCT('Slotted Extrusion - 20 x 20 x 400 mm',
'Slotted Extrusion - 20 x 20 x 400 mm',
'Slotted Extrusion - 20 x 20 x 400 mm',(#44065));
#44182=COLOUR_RGB('Light Blue',0.38,0.62,0.78);
#44183=FILL_AREA_STYLE_COLOUR('',#44182);
#44184=FILL_AREA_STYLE('',(#44183));
#44185=SURFACE_STYLE_FILL_AREA(#44184);
#44186=SURFACE_SIDE_STYLE('',(#44185));
#44187=SURFACE_STYLE_USAGE(.BOTH.,#44186);
#44188=PRESENTATION_STYLE_ASSIGNMENT((#44187));
ENDSEC;
END-ISO-10303-21;
